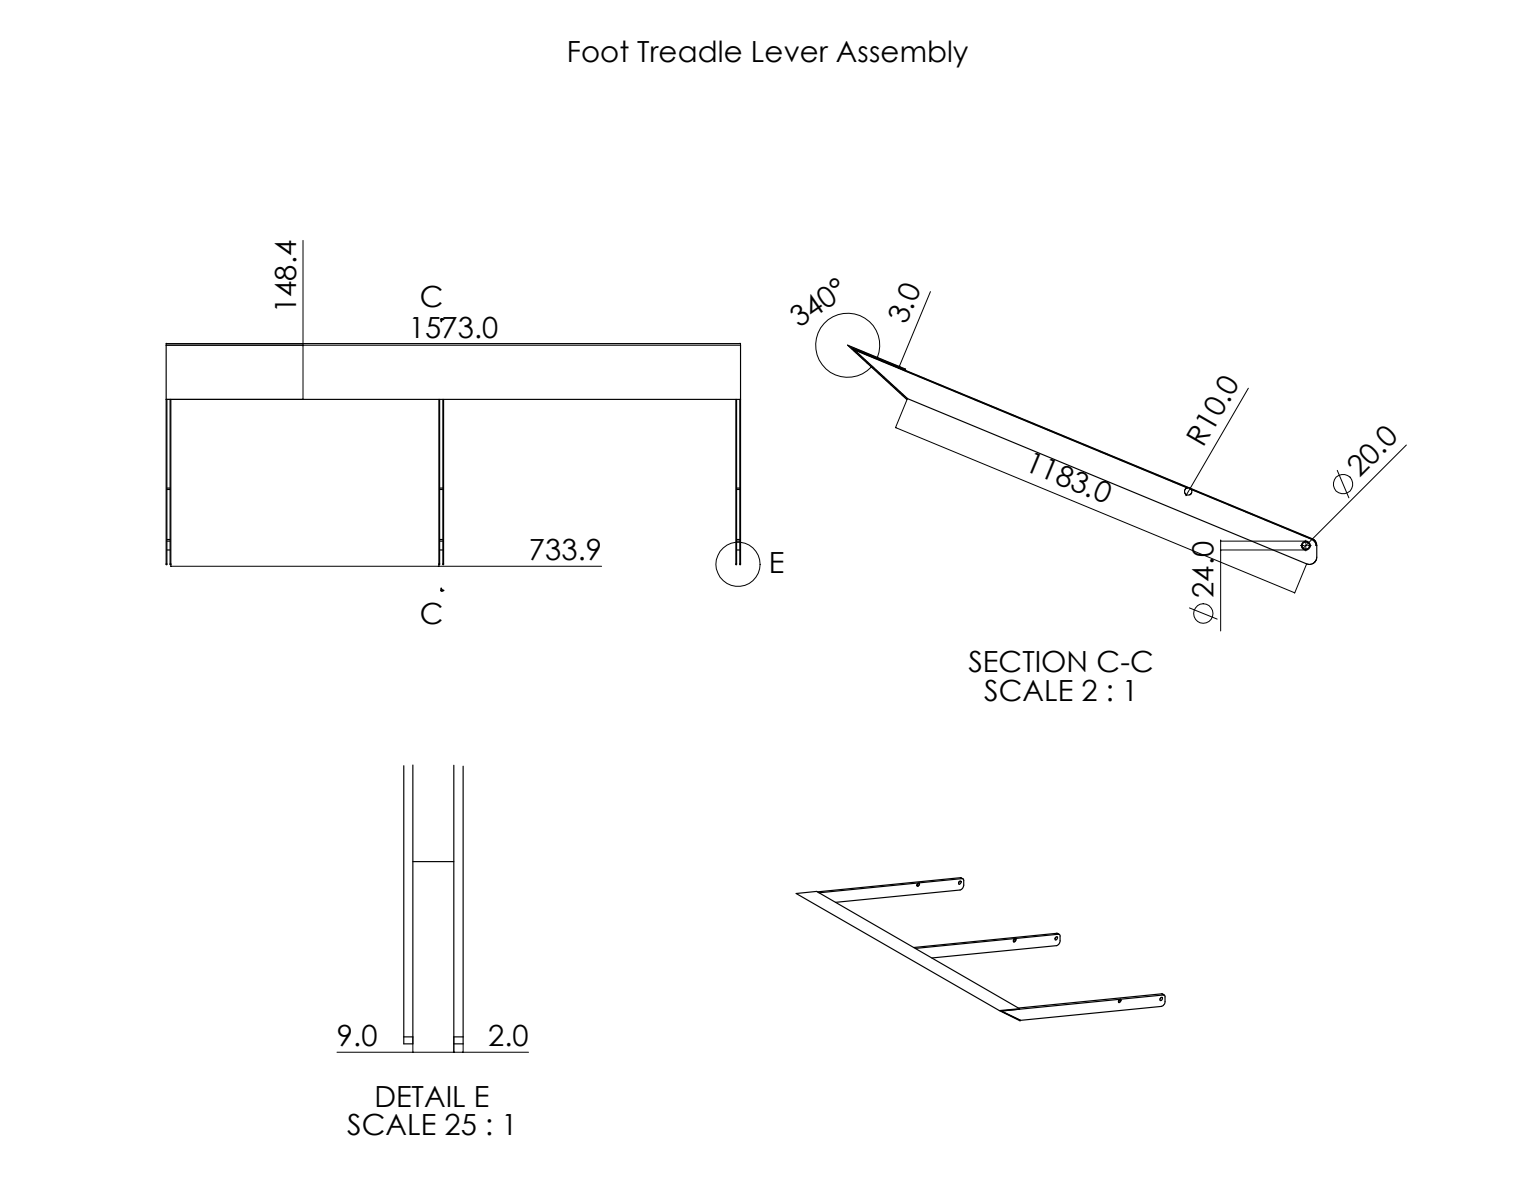
ISO-10303-21;
HEADER;
FILE_DESCRIPTION (('STEP AP214'),
    '1' );
FILE_NAME ('Foot Treadle Lever Assembly.step',
    '2026-10-21T17:07:05',
    ( '' ),
    ( '' ),
    'SwSTEP 2.0',
    'SolidWorks 2025',
    '' );
FILE_SCHEMA (( 'AUTOMOTIVE_DESIGN' ));
ENDSEC;

DATA;
#11=LINE ( 'NONE', #39516, #42666 ) ;
#12=ORIENTED_EDGE ( 'NONE', *, *, #22946, .T. ) ;
#20=ORIENTED_EDGE ( 'NONE', *, *, #3532, .T. ) ;
#69=VERTEX_POINT ( 'NONE', #2595 ) ;
#77=CARTESIAN_POINT ( 'NONE',  ( -39.63011601220123481, -365.3551492539851893, -28.13243251470704109 ) ) ;
#132=EDGE_CURVE ( 'NONE', #43251, #1390, #14358, .T. ) ;
#144=CARTESIAN_POINT ( 'NONE',  ( -786.4999999999993179, -512.9681489794448908, -339.9999999999999432 ) ) ;
#161=LINE ( 'NONE', #18412, #9196 ) ;
#169=EDGE_CURVE ( 'NONE', #1813, #29494, #23376, .T. ) ;
#171=ORIENTED_EDGE ( 'NONE', *, *, #19921, .T. ) ;
#197=CARTESIAN_POINT ( 'NONE',  ( 784.4999999999993179, -513.1383975375929367, -369.9999999999999432 ) ) ;
#209=PLANE ( 'NONE',  #44022 ) ;
#214=AXIS2_PLACEMENT_3D ( 'NONE', #42407, #11013, #31569 ) ;
#235=ORIENTED_EDGE ( 'NONE', *, *, #15168, .F. ) ;
#247=CARTESIAN_POINT ( 'NONE',  ( 775.4999999999993179, -544.8427095258973623, -350.0000000000000000 ) ) ;
#258=VECTOR ( 'NONE', #1525, 1000.000000000000000 ) ;
#260=LINE ( 'NONE', #35579, #37744 ) ;
#292=ORIENTED_EDGE ( 'NONE', *, *, #37389, .F. ) ;
#309=ORIENTED_EDGE ( 'NONE', *, *, #5989, .F. ) ;
#312=FACE_OUTER_BOUND ( 'NONE', #6954, .T. ) ;
#315=DIRECTION ( 'NONE',  ( 0.000000000000000000, 1.000000000000000000, -0.000000000000000000 ) ) ;
#317=EDGE_CURVE ( 'NONE', #3483, #7856, #33327, .T. ) ;
#318=DIRECTION ( 'NONE',  ( 0.000000000000000000, 0.000000000000000000, 1.000000000000000000 ) ) ;
#348=AXIS2_PLACEMENT_3D ( 'NONE', #27817, #38919, #20427 ) ;
#357=ORIENTED_EDGE ( 'NONE', *, *, #4281, .F. ) ;
#384=FACE_OUTER_BOUND ( 'NONE', #6648, .T. ) ;
#385=DIRECTION ( 'NONE',  ( -0.000000000000000000, -0.3826834323650838976, -0.9238795325112892920 ) ) ;
#415=EDGE_LOOP ( 'NONE', ( #32873, #15091, #12065, #25455 ) ) ;
#427=DIRECTION ( 'NONE',  ( 0.000000000000000000, 0.000000000000000000, 1.000000000000000000 ) ) ;
#463=VERTEX_POINT ( 'NONE', #38172 ) ;
#480=EDGE_LOOP ( 'NONE', ( #309, #39907, #31918, #2309 ) ) ;
#501=CARTESIAN_POINT ( 'NONE',  ( -39.63011601220123481, -563.3203001761230553, -342.3463313526983143 ) ) ;
#503=CARTESIAN_POINT ( 'NONE',  ( -773.4999999999993179, -512.9681489794448908, -339.9999999999999432 ) ) ;
#518=VERTEX_POINT ( 'NONE', #16922 ) ;
#526=CARTESIAN_POINT ( 'NONE',  ( 786.4999999999993179, -494.6608068873671300, -357.6536686473015720 ) ) ;
#552=VECTOR ( 'NONE', #9585, 1000.000000000000000 ) ;
#573=CARTESIAN_POINT ( 'NONE',  ( -773.4999999999993179, -365.3551492539851893, -28.13243251470704109 ) ) ;
#598=CARTESIAN_POINT ( 'NONE',  ( -786.4999999999993179, -544.8427095258973623, -350.0000000000000000 ) ) ;
#601=VERTEX_POINT ( 'NONE', #17377 ) ;
#603=CARTESIAN_POINT ( 'NONE',  ( 775.4999999999993179, 22.32581219114657856, 895.6886905569881492 ) ) ;
#611=CARTESIAN_POINT ( 'NONE',  ( 775.4999999999993179, -365.3551492539851893, -18.13243251470705886 ) ) ;
#612=FACE_OUTER_BOUND ( 'NONE', #6643, .T. ) ;
#628=AXIS2_PLACEMENT_3D ( 'NONE', #31793, #14497, #10794 ) ;
#630=PLANE ( 'NONE',  #9977 ) ;
#645=SHAPE_DEFINITION_REPRESENTATION ( #14496, #4721 ) ;
#656=FACE_OUTER_BOUND ( 'NONE', #25655, .T. ) ;
#661=DIRECTION ( 'NONE',  ( -1.000000000000000000, -0.000000000000000000, -0.000000000000000000 ) ) ;
#694=ORIENTED_EDGE ( 'NONE', *, *, #17918, .T. ) ;
#749=ORIENTED_EDGE ( 'NONE', *, *, #32375, .T. ) ;
#757=VERTEX_POINT ( 'NONE', #11595 ) ;
#764=ORIENTED_EDGE ( 'NONE', *, *, #41585, .T. ) ;
#790=DIRECTION ( 'NONE',  ( -1.000000000000000000, -0.000000000000000000, -0.000000000000000000 ) ) ;
#835=CARTESIAN_POINT ( 'NONE',  ( -786.4999999999993179, -544.8427095258973623, -350.0000000000000000 ) ) ;
#842=CYLINDRICAL_SURFACE ( 'NONE', #628, 12.00000000000001066 ) ;
#871=DIRECTION ( 'NONE',  ( 1.000000000000000000, -0.000000000000000000, -0.000000000000000000 ) ) ;
#877=CARTESIAN_POINT ( 'NONE',  ( -37.63011601220122770, -365.3551492539851893, -18.13243251470705886 ) ) ;
#909=CIRCLE ( 'NONE', #14943, 12.00000000000001066 ) ;
#964=VECTOR ( 'NONE', #44223, 999.9999999999998863 ) ;
#968=ORIENTED_EDGE ( 'NONE', *, *, #23222, .T. ) ;
#988=EDGE_CURVE ( 'NONE', #30488, #37811, #44694, .T. ) ;
#993=CARTESIAN_POINT ( 'NONE',  ( -39.63011601220123481, 26.27639943461401018, 900.0000000000001137 ) ) ;
#1012=CYLINDRICAL_SURFACE ( 'NONE', #8516, 19.99999999999990763 ) ;
#1029=VERTEX_POINT ( 'NONE', #23428 ) ;
#1033=VECTOR ( 'NONE', #41918, 1000.000000000000000 ) ;
#1058=CARTESIAN_POINT ( 'NONE',  ( -39.63011601220123481, -513.1383975375929367, -369.9999999999999432 ) ) ;
#1064=CARTESIAN_POINT ( 'NONE',  ( 775.4999999999993179, -544.8427095258973623, -369.9999999999999432 ) ) ;
#1101=PLANE ( 'NONE',  #32125 ) ;
#1103=AXIS2_PLACEMENT_3D ( 'NONE', #14608, #33065, #18972 ) ;
#1111=VERTEX_POINT ( 'NONE', #27142 ) ;
#1114=CARTESIAN_POINT ( 'NONE',  ( 746.4999999999993179, -355.4967352946684969, -16.45562775363632113 ) ) ;
#1131=ADVANCED_FACE ( 'NONE', ( #12811 ), #6108, .T. ) ;
#1132=AXIS2_PLACEMENT_3D ( 'NONE', #28850, #42931, #11297 ) ;
#1138=ORIENTED_EDGE ( 'NONE', *, *, #33206, .F. ) ;
#1159=LINE ( 'NONE', #8320, #2670 ) ;
#1203=AXIS2_PLACEMENT_3D ( 'NONE', #24325, #16957, #10469 ) ;
#1206=ORIENTED_EDGE ( 'NONE', *, *, #37580, .T. ) ;
#1219=ORIENTED_EDGE ( 'NONE', *, *, #41907, .T. ) ;
#1238=AXIS2_PLACEMENT_3D ( 'NONE', #7481, #21783, #18105 ) ;
#1240=LINE ( 'NONE', #4488, #19538 ) ;
#1243=AXIS2_PLACEMENT_3D ( 'NONE', #9404, #29728, #29961 ) ;
#1259=ORIENTED_EDGE ( 'NONE', *, *, #45039, .T. ) ;
#1266=EDGE_CURVE ( 'NONE', #33715, #16430, #19508, .T. ) ;
#1289=FACE_OUTER_BOUND ( 'NONE', #14899, .T. ) ;
#1320=ORIENTED_EDGE ( 'NONE', *, *, #28389, .T. ) ;
#1360=ORIENTED_EDGE ( 'NONE', *, *, #33421, .T. ) ;
#1374=VERTEX_POINT ( 'NONE', #10723 ) ;
#1376=VECTOR ( 'NONE', #35836, 999.9999999999998863 ) ;
#1390=VERTEX_POINT ( 'NONE', #6570 ) ;
#1418=MANIFOLD_SOLID_BREP ( 'Mirror5[3]', #38730 ) ;
#1429=VERTEX_POINT ( 'NONE', #2881 ) ;
#1440=DIRECTION ( 'NONE',  ( 0.000000000000000000, 0.000000000000000000, 1.000000000000000000 ) ) ;
#1480=ORIENTED_EDGE ( 'NONE', *, *, #43372, .T. ) ;
#1487=EDGE_CURVE ( 'NONE', #36764, #29494, #41917, .T. ) ;
#1490=DIRECTION ( 'NONE',  ( 0.000000000000000000, 0.000000000000000000, -1.000000000000000000 ) ) ;
#1499=PLANE ( 'NONE',  #38589 ) ;
#1517=FACE_BOUND ( 'NONE', #4195, .T. ) ;
#1525=DIRECTION ( 'NONE',  ( 1.000000000000000000, -0.000000000000000000, -0.000000000000000000 ) ) ;
#1530=ADVANCED_FACE ( 'NONE', ( #14425 ), #42133, .F. ) ;
#1535=ORIENTED_EDGE ( 'NONE', *, *, #32375, .F. ) ;
#1556=ORIENTED_EDGE ( 'NONE', *, *, #21278, .F. ) ;
#1559=DIRECTION ( 'NONE',  ( 1.000000000000000000, 0.000000000000000000, -0.000000000000000000 ) ) ;
#1640=ORIENTED_EDGE ( 'NONE', *, *, #30606, .T. ) ;
#1655=LINE ( 'NONE', #33102, #38693 ) ;
#1705=CIRCLE ( 'NONE', #44413, 12.00000000000001066 ) ;
#1718=CARTESIAN_POINT ( 'NONE',  ( 773.4999999999993179, -110.5936016518799221, 750.6326042729449455 ) ) ;
#1734=ORIENTED_EDGE ( 'NONE', *, *, #8319, .T. ) ;
#1743=ORIENTED_EDGE ( 'NONE', *, *, #15407, .F. ) ;
#1755=DIRECTION ( 'NONE',  ( 0.000000000000000000, 0.7372773368101328550, -0.6755902076156506952 ) ) ;
#1763=DIRECTION ( 'NONE',  ( -1.000000000000000000, -0.000000000000000000, -0.000000000000000000 ) ) ;
#1776=EDGE_CURVE ( 'NONE', #14297, #8747, #14884, .T. ) ;
#1795=ORIENTED_EDGE ( 'NONE', *, *, #40528, .F. ) ;
#1800=DIRECTION ( 'NONE',  ( 0.000000000000000000, 0.3826834323650836756, 0.9238795325112892920 ) ) ;
#1813=VERTEX_POINT ( 'NONE', #33115 ) ;
#1816=ORIENTED_EDGE ( 'NONE', *, *, #41907, .F. ) ;
#1833=CARTESIAN_POINT ( 'NONE',  ( -786.4999999999993179, -365.3551492539851893, -8.132432514707076621 ) ) ;
#1867=ORIENTED_EDGE ( 'NONE', *, *, #39030, .T. ) ;
#1888=DIRECTION ( 'NONE',  ( 0.000000000000000000, 0.3826834323650836756, 0.9238795325112892920 ) ) ;
#1893=VECTOR ( 'NONE', #35927, 1000.000000000000114 ) ;
#1895=DIRECTION ( 'NONE',  ( 0.000000000000000000, 0.000000000000000000, 1.000000000000000000 ) ) ;
#1921=ORIENTED_EDGE ( 'NONE', *, *, #37141, .F. ) ;
#1923=VECTOR ( 'NONE', #5270, 1000.000000000000114 ) ;
#1925=( NAMED_UNIT ( * ) SI_UNIT ( $, .STERADIAN. ) SOLID_ANGLE_UNIT ( ) );
#1926=AXIS2_PLACEMENT_3D ( 'NONE', #2058, #12918, #37160 ) ;
#1959=DIRECTION ( 'NONE',  ( 0.000000000000000000, -0.3826834323650836756, -0.9238795325112892920 ) ) ;
#1991=AXIS2_PLACEMENT_3D ( 'NONE', #31297, #3813, #21817 ) ;
#1996=CIRCLE ( 'NONE', #10121, 9.999999999999982236 ) ;
#1998=DIRECTION ( 'NONE',  ( 1.000000000000000000, 0.000000000000000000, -0.000000000000000000 ) ) ;
#2008=CARTESIAN_POINT ( 'NONE',  ( -28.63011601220122415, -501.1515549466498669, -368.0974687824633520 ) ) ;
#2030=ADVANCED_FACE ( 'NONE', ( #37471 ), #16221, .F. ) ;
#2041=ORIENTED_EDGE ( 'NONE', *, *, #11895, .F. ) ;
#2056=AXIS2_PLACEMENT_3D ( 'NONE', #19204, #36975, #15306 ) ;
#2058=CARTESIAN_POINT ( 'NONE',  ( -786.4999999999993179, -512.9681489794448908, -339.9999999999999432 ) ) ;
#2064=VERTEX_POINT ( 'NONE', #22914 ) ;
#2085=ADVANCED_FACE ( 'NONE', ( #40494 ), #20136, .T. ) ;
#2103=VERTEX_POINT ( 'NONE', #5150 ) ;
#2118=DIRECTION ( 'NONE',  ( 0.000000000000000000, 0.000000000000000000, -1.000000000000000000 ) ) ;
#2163=EDGE_LOOP ( 'NONE', ( #2260, #40842 ) ) ;
#2171=VERTEX_POINT ( 'NONE', #27982 ) ;
#2173=FACE_OUTER_BOUND ( 'NONE', #43522, .T. ) ;
#2175=EDGE_LOOP ( 'NONE', ( #2685, #9652 ) ) ;
#2190=DIRECTION ( 'NONE',  ( -1.000000000000000000, -0.000000000000000000, -0.000000000000000000 ) ) ;
#2212=ORIENTED_EDGE ( 'NONE', *, *, #10099, .F. ) ;
#2217=ORIENTED_EDGE ( 'NONE', *, *, #15681, .F. ) ;
#2219=ORIENTED_EDGE ( 'NONE', *, *, #36874, .F. ) ;
#2247=ORIENTED_EDGE ( 'NONE', *, *, #26936, .F. ) ;
#2257=CARTESIAN_POINT ( 'NONE',  ( -28.63011601220122415, -857.0166862835568509, -63.94525337997358605 ) ) ;
#2260=ORIENTED_EDGE ( 'NONE', *, *, #28130, .F. ) ;
#2273=VERTEX_POINT ( 'NONE', #44865 ) ;
#2291=LINE ( 'NONE', #22859, #8243 ) ;
#2309=ORIENTED_EDGE ( 'NONE', *, *, #15175, .T. ) ;
#2313=EDGE_CURVE ( 'NONE', #30501, #26595, #11394, .T. ) ;
#2326=ORIENTED_EDGE ( 'NONE', *, *, #36268, .T. ) ;
#2367=EDGE_CURVE ( 'NONE', #2677, #39212, #37185, .T. ) ;
#2381=EDGE_LOOP ( 'NONE', ( #23102, #23854, #14000, #2217, #1867, #3901, #27773, #25609, #12738, #13022, #39635, #33451 ) ) ;
#2388=CARTESIAN_POINT ( 'NONE',  ( 786.4999999999993179, -512.9681489794448908, -339.9999999999999432 ) ) ;
#2391=EDGE_LOOP ( 'NONE', ( #6090, #18144, #8044, #23562 ) ) ;
#2408=CARTESIAN_POINT ( 'NONE',  ( -66.63011601220125613, -359.5698779088871788, -26.28906389436294688 ) ) ;
#2413=DIRECTION ( 'NONE',  ( 1.000000000000000000, -0.000000000000000000, -0.000000000000000000 ) ) ;
#2426=CARTESIAN_POINT ( 'NONE',  ( -26.63011601220122060, -544.8427095258973623, -369.9999999999999432 ) ) ;
#2442=CIRCLE ( 'NONE', #9836, 9.999999999999980460 ) ;
#2451=CARTESIAN_POINT ( 'NONE',  ( 784.4999999999993179, -544.8427095258973623, -369.9999999999999432 ) ) ;
#2460=CARTESIAN_POINT ( 'NONE',  ( 773.4999999999993179, -513.1383975375929367, -369.9999999999999432 ) ) ;
#2463=LINE ( 'NONE', #29964, #24876 ) ;
#2472=DIRECTION ( 'NONE',  ( -1.000000000000000000, -0.000000000000000000, -0.000000000000000000 ) ) ;
#2475=AXIS2_PLACEMENT_3D ( 'NONE', #835, #35477, #7779 ) ;
#2495=VERTEX_POINT ( 'NONE', #18057 ) ;
#2505=AXIS2_PLACEMENT_3D ( 'NONE', #7274, #13509, #10484 ) ;
#2507=ORIENTED_EDGE ( 'NONE', *, *, #20142, .T. ) ;
#2526=AXIS2_PLACEMENT_3D ( 'NONE', #30837, #37766, #6115 ) ;
#2529=FACE_OUTER_BOUND ( 'NONE', #15063, .T. ) ;
#2561=ORIENTED_EDGE ( 'NONE', *, *, #11429, .F. ) ;
#2587=CARTESIAN_POINT ( 'NONE',  ( 1007.605605532488426, -295.7697417039441916, 122.5118383533586837 ) ) ;
#2590=DIRECTION ( 'NONE',  ( 0.000000000000000000, 0.000000000000000000, -1.000000000000000000 ) ) ;
#2595=CARTESIAN_POINT ( 'NONE',  ( -773.4999999999993179, -563.3203001761230553, -342.3463313526983143 ) ) ;
#2609=CIRCLE ( 'NONE', #10002, 9.999999999999982236 ) ;
#2614=VECTOR ( 'NONE', #34560, 1000.000000000000000 ) ;
#2615=ORIENTED_EDGE ( 'NONE', *, *, #30089, .T. ) ;
#2634=LINE ( 'NONE', #19962, #23991 ) ;
#2635=DIRECTION ( 'NONE',  ( -1.000000000000000000, -0.000000000000000000, 0.000000000000000000 ) ) ;
#2651=CARTESIAN_POINT ( 'NONE',  ( -773.4999999999993179, -513.1383975375929367, -349.9999999999999432 ) ) ;
#2670=VECTOR ( 'NONE', #22384, 1000.000000000000114 ) ;
#2677=VERTEX_POINT ( 'NONE', #21737 ) ;
#2685=ORIENTED_EDGE ( 'NONE', *, *, #32862, .T. ) ;
#2700=FACE_OUTER_BOUND ( 'NONE', #35564, .T. ) ;
#2708=EDGE_CURVE ( 'NONE', #5066, #9279, #9897, .T. ) ;
#2716=CARTESIAN_POINT ( 'NONE',  ( -37.63011601220122770, -544.8427095258973623, -350.0000000000000000 ) ) ;
#2731=CIRCLE ( 'NONE', #18210, 10.00000000000000888 ) ;
#2753=CIRCLE ( 'NONE', #18985, 10.00000000000000888 ) ;
#2796=CARTESIAN_POINT ( 'NONE',  ( -26.63011601220122060, -110.5936016518799221, 750.6326042729449455 ) ) ;
#2824=DIRECTION ( 'NONE',  ( -1.000000000000000000, -0.000000000000000000, 0.000000000000000000 ) ) ;
#2847=ORIENTED_EDGE ( 'NONE', *, *, #24646, .T. ) ;
#2856=CIRCLE ( 'NONE', #24244, 9.999999999999980460 ) ;
#2863=ORIENTED_EDGE ( 'NONE', *, *, #5989, .T. ) ;
#2866=CARTESIAN_POINT ( 'NONE',  ( 746.4999999999993179, -365.3551492539851893, -8.132432514707076621 ) ) ;
#2875=CARTESIAN_POINT ( 'NONE',  ( -775.4999999999993179, -365.3551492539851893, -18.13243251470705886 ) ) ;
#2881=CARTESIAN_POINT ( 'NONE',  ( 775.4999999999993179, -563.3203001761230553, -342.3463313526983143 ) ) ;
#2892=CIRCLE ( 'NONE', #14720, 12.00000000000001066 ) ;
#2897=ORIENTED_EDGE ( 'NONE', *, *, #38295, .F. ) ;
#2902=CARTESIAN_POINT ( 'NONE',  ( 786.4999999999993179, -496.5085659523897448, -356.8883017825714319 ) ) ;
#2912=ORIENTED_EDGE ( 'NONE', *, *, #37065, .T. ) ;
#2918=CARTESIAN_POINT ( 'NONE',  ( -26.63011601220122060, -512.9681489794448908, -352.0000000000000000 ) ) ;
#2932=DIRECTION ( 'NONE',  ( -0.000000000000000000, 1.000000000000000000, -0.000000000000000000 ) ) ;
#2937=CARTESIAN_POINT ( 'NONE',  ( 786.4999999999993179, -365.3551492539851893, -8.132432514707076621 ) ) ;
#2943=ORIENTED_EDGE ( 'NONE', *, *, #32872, .T. ) ;
#2947=EDGE_CURVE ( 'NONE', #11840, #5018, #12035, .T. ) ;
#2950=CARTESIAN_POINT ( 'NONE',  ( -786.4999999999993179, -494.6608068873671300, -357.6536686473015720 ) ) ;
#2955=CARTESIAN_POINT ( 'NONE',  ( -39.63011601220123481, -512.9681489794448908, -339.9999999999999432 ) ) ;
#2958=VERTEX_POINT ( 'NONE', #33493 ) ;
#3021=LINE ( 'NONE', #2796, #39689 ) ;
#3085=DIRECTION ( 'NONE',  ( 1.000000000000000000, 0.000000000000000000, -0.000000000000000000 ) ) ;
#3086=LINE ( 'NONE', #2866, #40334 ) ;
#3089=VECTOR ( 'NONE', #24966, 1000.000000000000000 ) ;
#3121=FACE_OUTER_BOUND ( 'NONE', #37828, .T. ) ;
#3143=AXIS2_PLACEMENT_3D ( 'NONE', #45436, #38276, #45669 ) ;
#3146=CYLINDRICAL_SURFACE ( 'NONE', #3469, 10.00000000000000888 ) ;
#3152=DIRECTION ( 'NONE',  ( -1.000000000000000000, -0.000000000000000000, -0.000000000000000000 ) ) ;
#3157=DIRECTION ( 'NONE',  ( -1.000000000000000000, -0.000000000000000000, -0.000000000000000000 ) ) ;
#3169=DIRECTION ( 'NONE',  ( -1.000000000000000000, 0.000000000000000000, 0.000000000000000000 ) ) ;
#3174=DIRECTION ( 'NONE',  ( 0.000000000000000000, 0.000000000000000000, -1.000000000000000000 ) ) ;
#3186=ORIENTED_EDGE ( 'NONE', *, *, #45316, .T. ) ;
#3187=AXIS2_PLACEMENT_3D ( 'NONE', #13354, #45692, #3174 ) ;
#3201=CARTESIAN_POINT ( 'NONE',  ( 786.4999999999993179, -544.8427095258973623, -369.9999999999999432 ) ) ;
#3219=CIRCLE ( 'NONE', #24604, 18.00000000000001421 ) ;
#3263=DIRECTION ( 'NONE',  ( -1.000000000000000000, -0.000000000000000000, 0.000000000000000000 ) ) ;
#3293=ORIENTED_EDGE ( 'NONE', *, *, #27744, .F. ) ;
#3312=ORIENTED_EDGE ( 'NONE', *, *, #8604, .F. ) ;
#3315=AXIS2_PLACEMENT_3D ( 'NONE', #45042, #34639, #16633 ) ;
#3320=MANIFOLD_SOLID_BREP ( 'Cut-Extrude8', #6229 ) ;
#3337=AXIS2_PLACEMENT_3D ( 'NONE', #41849, #38377, #14122 ) ;
#3342=( NAMED_UNIT ( * ) PLANE_ANGLE_UNIT ( ) SI_UNIT ( $, .RADIAN. ) );
#3376=ORIENTED_EDGE ( 'NONE', *, *, #23841, .T. ) ;
#3451=AXIS2_PLACEMENT_3D ( 'NONE', #42334, #21326, #31709 ) ;
#3469=AXIS2_PLACEMENT_3D ( 'NONE', #144, #6618, #38485 ) ;
#3483=VERTEX_POINT ( 'NONE', #18684 ) ;
#3497=CARTESIAN_POINT ( 'NONE',  ( -786.4999999999993179, -110.5936016518799221, 750.6326042729449455 ) ) ;
#3499=DIRECTION ( 'NONE',  ( 1.000000000000000000, 0.000000000000000000, -0.000000000000000000 ) ) ;
#3511=DIRECTION ( 'NONE',  ( 0.000000000000000000, 0.000000000000000000, -1.000000000000000000 ) ) ;
#3517=DIRECTION ( 'NONE',  ( 0.000000000000000000, 0.000000000000000000, 1.000000000000000000 ) ) ;
#3532=EDGE_CURVE ( 'NONE', #35031, #33715, #11535, .T. ) ;
#3533=CARTESIAN_POINT ( 'NONE',  ( -786.4999999999993179, -513.1383975375929367, -369.9999999999999432 ) ) ;
#3542=VERTEX_POINT ( 'NONE', #21927 ) ;
#3545=PLANE ( 'NONE',  #24184 ) ;
#3550=ADVANCED_FACE ( 'NONE', ( #25617 ), #32324, .T. ) ;
#3561=DIRECTION ( 'NONE',  ( 1.000000000000000000, -0.000000000000000000, -0.000000000000000000 ) ) ;
#3601=CARTESIAN_POINT ( 'NONE',  ( -28.63011601220122415, -563.3203001761231690, -342.3463313526983143 ) ) ;
#3612=VERTEX_POINT ( 'NONE', #23552 ) ;
#3616=DIRECTION ( 'NONE',  ( 0.000000000000000000, 0.000000000000000000, 1.000000000000000000 ) ) ;
#3642=CARTESIAN_POINT ( 'NONE',  ( -26.63011601220122060, -365.3551492539851893, -8.132432514707076621 ) ) ;
#3648=LINE ( 'NONE', #7110, #17334 ) ;
#3705=ORIENTED_EDGE ( 'NONE', *, *, #17646, .F. ) ;
#3726=ORIENTED_EDGE ( 'NONE', *, *, #27806, .F. ) ;
#3741=CARTESIAN_POINT ( 'NONE',  ( -37.63011601220122770, -512.9681489794448908, -352.0000000000000000 ) ) ;
#3768=ORIENTED_EDGE ( 'NONE', *, *, #28665, .F. ) ;
#3776=ORIENTED_EDGE ( 'NONE', *, *, #45342, .T. ) ;
#3799=EDGE_CURVE ( 'NONE', #36535, #14349, #2609, .T. ) ;
#3800=LINE ( 'NONE', #28968, #14383 ) ;
#3809=ORIENTED_EDGE ( 'NONE', *, *, #12744, .F. ) ;
#3813=DIRECTION ( 'NONE',  ( -1.000000000000000000, 0.000000000000000000, 0.000000000000000000 ) ) ;
#3818=ADVANCED_FACE ( 'NONE', ( #40894 ), #12490, .F. ) ;
#3837=CARTESIAN_POINT ( 'NONE',  ( -784.4999999999993179, -544.8427095258973623, -350.0000000000000000 ) ) ;
#3860=CARTESIAN_POINT ( 'NONE',  ( -784.4999999999993179, -365.3551492539851893, -18.13243251470705886 ) ) ;
#3870=CYLINDRICAL_SURFACE ( 'NONE', #3187, 9.999999999999980460 ) ;
#3876=VECTOR ( 'NONE', #8066, 1000.000000000000000 ) ;
#3891=DIRECTION ( 'NONE',  ( 0.000000000000000000, 0.000000000000000000, 1.000000000000000000 ) ) ;
#3901=ORIENTED_EDGE ( 'NONE', *, *, #6862, .T. ) ;
#3941=VECTOR ( 'NONE', #43200, 1000.000000000000000 ) ;
#3965=CARTESIAN_POINT ( 'NONE',  ( 786.4999999999993179, -544.8427095258973623, -369.9999999999999432 ) ) ;
#4005=FACE_OUTER_BOUND ( 'NONE', #18702, .T. ) ;
#4006=AXIS2_PLACEMENT_3D ( 'NONE', #9807, #34741, #34279 ) ;
#4041=VECTOR ( 'NONE', #22643, 1000.000000000000114 ) ;
#4047=VECTOR ( 'NONE', #8844, 1000.000000000000000 ) ;
#4067=VERTEX_POINT ( 'NONE', #29061 ) ;
#4073=CARTESIAN_POINT ( 'NONE',  ( 746.4999999999993179, -365.3551492539851893, -18.13243251470705886 ) ) ;
#4084=ADVANCED_FACE ( 'NONE', ( #10827, #656, #18227 ), #25354, .F. ) ;
#4119=VECTOR ( 'NONE', #8933, 1000.000000000000000 ) ;
#4136=CIRCLE ( 'NONE', #36560, 12.00000000000001066 ) ;
#4161=VECTOR ( 'NONE', #30084, 1000.000000000000114 ) ;
#4169=ADVANCED_FACE ( 'NONE', ( #32754 ), #1101, .T. ) ;
#4186=ORIENTED_EDGE ( 'NONE', *, *, #41613, .F. ) ;
#4195=EDGE_LOOP ( 'NONE', ( #34713, #2219 ) ) ;
#4226=ORIENTED_EDGE ( 'NONE', *, *, #132, .T. ) ;
#4245=ORIENTED_EDGE ( 'NONE', *, *, #4281, .T. ) ;
#4270=DIRECTION ( 'NONE',  ( -1.000000000000000000, -0.000000000000000000, -0.000000000000000000 ) ) ;
#4271=ORIENTED_EDGE ( 'NONE', *, *, #20771, .T. ) ;
#4275=DIRECTION ( 'NONE',  ( 1.000000000000000000, -0.000000000000000000, -0.000000000000000000 ) ) ;
#4281=EDGE_CURVE ( 'NONE', #33261, #44892, #11744, .T. ) ;
#4297=CARTESIAN_POINT ( 'NONE',  ( 773.4999999999993179, -544.8427095258973623, -369.9999999999999432 ) ) ;
#4300=ORIENTED_EDGE ( 'NONE', *, *, #37389, .T. ) ;
#4309=LINE ( 'NONE', #11695, #44390 ) ;
#4320=EDGE_CURVE ( 'NONE', #14349, #36535, #20311, .T. ) ;
#4326=AXIS2_PLACEMENT_3D ( 'NONE', #28800, #38984, #43109 ) ;
#4358=VERTEX_POINT ( 'NONE', #23170 ) ;
#4382=ORIENTED_EDGE ( 'NONE', *, *, #14505, .T. ) ;
#4397=CARTESIAN_POINT ( 'NONE',  ( -786.4999999999993179, -496.5085659523897448, -356.8883017825714319 ) ) ;
#4398=ADVANCED_FACE ( 'NONE', ( #2173 ), #18900, .F. ) ;
#4401=EDGE_CURVE ( 'NONE', #13363, #45720, #2634, .T. ) ;
#4428=EDGE_CURVE ( 'NONE', #44892, #44015, #21080, .T. ) ;
#4454=VERTEX_POINT ( 'NONE', #37972 ) ;
#4467=CARTESIAN_POINT ( 'NONE',  ( 786.4999999999993179, 262.9227088301245203, 634.7515695135432452 ) ) ;
#4488=CARTESIAN_POINT ( 'NONE',  ( 786.4999999999993179, -110.5936016518799221, 750.6326042729449455 ) ) ;
#4529=FACE_OUTER_BOUND ( 'NONE', #29351, .T. ) ;
#4544=DIRECTION ( 'NONE',  ( -1.000000000000000000, -0.000000000000000000, -0.000000000000000000 ) ) ;
#4571=CARTESIAN_POINT ( 'NONE',  ( 775.4999999999993179, -365.3551492539851893, -28.13243251470704109 ) ) ;
#4577=DIRECTION ( 'NONE',  ( 1.000000000000000000, -0.000000000000000000, -0.000000000000000000 ) ) ;
#4580=LINE ( 'NONE', #26498, #3876 ) ;
#4607=ORIENTED_EDGE ( 'NONE', *, *, #43372, .F. ) ;
#4634=CARTESIAN_POINT ( 'NONE',  ( -26.63011601220122060, -513.1383975375929367, -349.9999999999999432 ) ) ;
#4642=EDGE_CURVE ( 'NONE', #6318, #39517, #7809, .T. ) ;
#4667=ORIENTED_EDGE ( 'NONE', *, *, #6862, .F. ) ;
#4703=VERTEX_POINT ( 'NONE', #24544 ) ;
#4721=SHAPE_REPRESENTATION ( 'Foot Treadle Lever Assembly', ( #26858 ), #34210 ) ;
#4722=EDGE_CURVE ( 'NONE', #42387, #22673, #38657, .T. ) ;
#4751=VECTOR ( 'NONE', #28100, 1000.000000000000000 ) ;
#4811=DIRECTION ( 'NONE',  ( 1.000000000000000000, -0.000000000000000000, -0.000000000000000000 ) ) ;
#4851=EDGE_LOOP ( 'NONE', ( #36463, #27555, #7077, #13940, #1219, #41795, #40284, #31017, #25069, #41649, #42787 ) ) ;
#4854=CARTESIAN_POINT ( 'NONE',  ( -66.63011601220125613, -365.3551492539851893, -18.13243251470705886 ) ) ;
#4891=EDGE_CURVE ( 'NONE', #1429, #37268, #16571, .T. ) ;
#4897=CIRCLE ( 'NONE', #14513, 9.999999999999982236 ) ;
#4914=ORIENTED_EDGE ( 'NONE', *, *, #13446, .T. ) ;
#4922=DIRECTION ( 'NONE',  ( 1.000000000000000000, 0.000000000000000000, -0.000000000000000000 ) ) ;
#4943=ORIENTED_EDGE ( 'NONE', *, *, #11926, .F. ) ;
#4962=VECTOR ( 'NONE', #41227, 1000.000000000000000 ) ;
#4980=DIRECTION ( 'NONE',  ( -1.000000000000000000, 0.000000000000000000, 0.000000000000000000 ) ) ;
#4988=ADVANCED_FACE ( 'NONE', ( #39819 ), #29407, .T. ) ;
#5012=AXIS2_PLACEMENT_3D ( 'NONE', #28929, #32405, #10686 ) ;
#5018=VERTEX_POINT ( 'NONE', #43479 ) ;
#5026=CARTESIAN_POINT ( 'NONE',  ( -786.4999999999993179, -512.9681489794448908, -329.9999999999999432 ) ) ;
#5056=CARTESIAN_POINT ( 'NONE',  ( 784.4999999999993179, -513.1383975375929367, -369.9999999999999432 ) ) ;
#5066=VERTEX_POINT ( 'NONE', #11847 ) ;
#5075=EDGE_LOOP ( 'NONE', ( #31549, #6184 ) ) ;
#5117=VERTEX_POINT ( 'NONE', #43700 ) ;
#5134=FACE_OUTER_BOUND ( 'NONE', #13937, .T. ) ;
#5150=CARTESIAN_POINT ( 'NONE',  ( -784.4999999999993179, -110.5936016518799221, 750.6326042729449455 ) ) ;
#5168=CARTESIAN_POINT ( 'NONE',  ( -37.63011601220122770, -496.5085659523897448, -356.8883017825714319 ) ) ;
#5182=EDGE_CURVE ( 'NONE', #36107, #601, #1655, .T. ) ;
#5248=LINE ( 'NONE', #40597, #11606 ) ;
#5270=DIRECTION ( 'NONE',  ( 0.000000000000000000, -0.6755902076156505842, -0.7372773368101327440 ) ) ;
#5337=EDGE_LOOP ( 'NONE', ( #40422, #292, #10993, #45248 ) ) ;
#5372=DIRECTION ( 'NONE',  ( -1.000000000000000000, -0.000000000000000000, -0.000000000000000000 ) ) ;
#5398=AXIS2_PLACEMENT_3D ( 'NONE', #4634, #6787, #18294 ) ;
#5426=CARTESIAN_POINT ( 'NONE',  ( -773.4999999999993179, -544.8427095258973623, -350.0000000000000000 ) ) ;
#5437=( NAMED_UNIT ( * ) PLANE_ANGLE_UNIT ( ) SI_UNIT ( $, .RADIAN. ) );
#5450=AXIS2_PLACEMENT_3D ( 'NONE', #19014, #12077, #36561 ) ;
#5518=ADVANCED_FACE ( 'NONE', ( #24914, #42024 ), #209, .T. ) ;
#5538=AXIS2_PLACEMENT_3D ( 'NONE', #14758, #21906, #427 ) ;
#5564=ORIENTED_EDGE ( 'NONE', *, *, #13446, .F. ) ;
#5577=ORIENTED_EDGE ( 'NONE', *, *, #10584, .T. ) ;
#5622=ORIENTED_EDGE ( 'NONE', *, *, #37385, .F. ) ;
#5655=LINE ( 'NONE', #2408, #22653 ) ;
#5658=CARTESIAN_POINT ( 'NONE',  ( -26.63011601220122060, -494.6608068873671300, -357.6536686473015720 ) ) ;
#5670=LINE ( 'NONE', #22978, #25449 ) ;
#5674=ORIENTED_EDGE ( 'NONE', *, *, #11458, .T. ) ;
#5708=FACE_OUTER_BOUND ( 'NONE', #31644, .T. ) ;
#5751=ORIENTED_EDGE ( 'NONE', *, *, #32627, .T. ) ;
#5782=LINE ( 'NONE', #16639, #13979 ) ;
#5817=EDGE_CURVE ( 'NONE', #4454, #22673, #29528, .T. ) ;
#5821=EDGE_CURVE ( 'NONE', #24190, #26595, #11969, .T. ) ;
#5831=CARTESIAN_POINT ( 'NONE',  ( -773.4999999999993179, -110.5936016518799221, 750.6326042729449455 ) ) ;
#5833=CARTESIAN_POINT ( 'NONE',  ( -26.63011601220122060, -494.6608068873671300, -357.6536686473015720 ) ) ;
#5836=CARTESIAN_POINT ( 'NONE',  ( 784.4999999999993179, 22.32581219114657856, 895.6886905569881492 ) ) ;
#5862=ORIENTED_EDGE ( 'NONE', *, *, #317, .T. ) ;
#5867=LINE ( 'NONE', #18037, #45475 ) ;
#5868=CARTESIAN_POINT ( 'NONE',  ( 773.4999999999993179, -513.1383975375929367, -349.9999999999999432 ) ) ;
#5872=CARTESIAN_POINT ( 'NONE',  ( -786.4999999999993179, -513.1383975375929367, -349.9999999999999432 ) ) ;
#5874=ORIENTED_EDGE ( 'NONE', *, *, #28330, .T. ) ;
#5877=DIRECTION ( 'NONE',  ( 0.000000000000000000, 0.3826834323650836756, 0.9238795325112892920 ) ) ;
#5915=EDGE_LOOP ( 'NONE', ( #33444, #35634, #11438, #18589 ) ) ;
#5927=DIRECTION ( 'NONE',  ( 0.000000000000000000, 1.000000000000000000, -0.000000000000000000 ) ) ;
#5936=CARTESIAN_POINT ( 'NONE',  ( 786.4999999999993179, -512.9681489794448908, -339.9999999999999432 ) ) ;
#5989=EDGE_CURVE ( 'NONE', #30700, #15113, #5655, .T. ) ;
#6009=EDGE_CURVE ( 'NONE', #17287, #23251, #2753, .T. ) ;
#6032=CARTESIAN_POINT ( 'NONE',  ( 784.4999999999993179, -365.3551492539851893, -28.13243251470704109 ) ) ;
#6053=DIRECTION ( 'NONE',  ( 0.000000000000000000, 0.000000000000000000, 1.000000000000000000 ) ) ;
#6060=EDGE_CURVE ( 'NONE', #22319, #19543, #16279, .T. ) ;
#6065=ADVANCED_FACE ( 'NONE', ( #23425 ), #30358, .F. ) ;
#6075=DIRECTION ( 'NONE',  ( 1.000000000000000000, 0.000000000000000000, 0.000000000000000000 ) ) ;
#6090=ORIENTED_EDGE ( 'NONE', *, *, #23320, .F. ) ;
#6101=CARTESIAN_POINT ( 'NONE',  ( -786.4999999999993179, -295.7697417039441916, 122.5118383533586837 ) ) ;
#6108=CYLINDRICAL_SURFACE ( 'NONE', #26110, 12.00000000000001066 ) ;
#6115=DIRECTION ( 'NONE',  ( 0.000000000000000000, 0.000000000000000000, 1.000000000000000000 ) ) ;
#6119=DIRECTION ( 'NONE',  ( -1.000000000000000000, 0.000000000000000000, 0.000000000000000000 ) ) ;
#6130=ORIENTED_EDGE ( 'NONE', *, *, #32264, .F. ) ;
#6138=ORIENTED_EDGE ( 'NONE', *, *, #35330, .F. ) ;
#6184=ORIENTED_EDGE ( 'NONE', *, *, #26462, .T. ) ;
#6229=CLOSED_SHELL ( 'NONE', ( #10346, #12867, #37117, #1530, #18516, #8801, #36126, #7214, #32583, #4084, #43045, #19268, #33761, #23580, #4988, #36322, #44499, #16813, #16830, #24365, #43560, #33510, #24320, #12302 ) ) ;
#6238=ORIENTED_EDGE ( 'NONE', *, *, #27806, .T. ) ;
#6241=UNCERTAINTY_MEASURE_WITH_UNIT (LENGTH_MEASURE( 1.000000000000000082E-05 ), #45148, 'distance_accuracy_value', 'NONE');
#6260=ORIENTED_EDGE ( 'NONE', *, *, #33421, .F. ) ;
#6276=ADVANCED_FACE ( 'NONE', ( #42130 ), #13506, .T. ) ;
#6318=VERTEX_POINT ( 'NONE', #17432 ) ;
#6342=EDGE_CURVE ( 'NONE', #4067, #1813, #42351, .T. ) ;
#6349=VECTOR ( 'NONE', #44431, 1000.000000000000000 ) ;
#6367=VECTOR ( 'NONE', #21963, 1000.000000000000000 ) ;
#6385=CIRCLE ( 'NONE', #3451, 19.99999999999990763 ) ;
#6481=ORIENTED_EDGE ( 'NONE', *, *, #37385, .T. ) ;
#6498=ORIENTED_EDGE ( 'NONE', *, *, #25485, .T. ) ;
#6503=ORIENTED_EDGE ( 'NONE', *, *, #10845, .T. ) ;
#6538=EDGE_LOOP ( 'NONE', ( #4300, #10500 ) ) ;
#6553=ORIENTED_EDGE ( 'NONE', *, *, #11895, .T. ) ;
#6570=CARTESIAN_POINT ( 'NONE',  ( -784.4999999999993179, -512.9681489794448908, -352.0000000000000000 ) ) ;
#6611=EDGE_CURVE ( 'NONE', #14349, #38546, #21561, .T. ) ;
#6618=DIRECTION ( 'NONE',  ( 1.000000000000000000, -0.000000000000000000, -0.000000000000000000 ) ) ;
#6633=DIRECTION ( 'NONE',  ( 0.000000000000000000, 0.3826834323650838421, 0.9238795325112891810 ) ) ;
#6641=DIRECTION ( 'NONE',  ( 0.000000000000000000, 0.000000000000000000, -1.000000000000000000 ) ) ;
#6643=EDGE_LOOP ( 'NONE', ( #35857, #18885, #44425, #10145 ) ) ;
#6648=EDGE_LOOP ( 'NONE', ( #32461, #24761, #13432, #33753 ) ) ;
#6670=CARTESIAN_POINT ( 'NONE',  ( 786.4999999999993179, -563.3203001761230553, -342.3463313526983143 ) ) ;
#6699=EDGE_LOOP ( 'NONE', ( #39109, #2326, #14048, #42847 ) ) ;
#6730=DIRECTION ( 'NONE',  ( 1.000000000000000000, -0.000000000000000000, -0.000000000000000000 ) ) ;
#6738=DIRECTION ( 'NONE',  ( 0.000000000000000000, 0.000000000000000000, 1.000000000000000000 ) ) ;
#6751=DIRECTION ( 'NONE',  ( 0.000000000000000000, 0.000000000000000000, 1.000000000000000000 ) ) ;
#6768=ORIENTED_EDGE ( 'NONE', *, *, #42448, .T. ) ;
#6774=CARTESIAN_POINT ( 'NONE',  ( 784.4999999999993179, -513.1383975375929367, -367.9999999999999432 ) ) ;
#6778=DIRECTION ( 'NONE',  ( 1.000000000000000000, 0.000000000000000000, 0.000000000000000000 ) ) ;
#6787=DIRECTION ( 'NONE',  ( -1.000000000000000000, -0.000000000000000000, -0.000000000000000000 ) ) ;
#6800=DIRECTION ( 'NONE',  ( 1.000000000000000000, 0.000000000000000000, -0.000000000000000000 ) ) ;
#6828=DIRECTION ( 'NONE',  ( -0.000000000000000000, -0.3826834323650838421, -0.9238795325112891810 ) ) ;
#6862=EDGE_CURVE ( 'NONE', #42371, #40010, #8571, .T. ) ;
#6878=AXIS2_PLACEMENT_3D ( 'NONE', #2955, #24878, #31803 ) ;
#6898=ORIENTED_EDGE ( 'NONE', *, *, #29198, .T. ) ;
#6902=VECTOR ( 'NONE', #40429, 1000.000000000000000 ) ;
#6908=EDGE_CURVE ( 'NONE', #1390, #6318, #25029, .T. ) ;
#6951=VECTOR ( 'NONE', #34287, 1000.000000000000000 ) ;
#6954=EDGE_LOOP ( 'NONE', ( #33679, #29390, #23621, #12123 ) ) ;
#6964=EDGE_CURVE ( 'NONE', #24418, #16954, #29854, .T. ) ;
#6987=DIRECTION ( 'NONE',  ( 0.000000000000000000, -0.9238795325112892920, 0.3826834323650836756 ) ) ;
#6998=DIRECTION ( 'NONE',  ( 0.000000000000000000, 0.6755902076156505842, 0.7372773368101327440 ) ) ;
#7004=CLOSED_SHELL ( 'NONE', ( #11735, #8851, #8351, #2085, #35382, #6276, #36538, #13914 ) ) ;
#7024=DIRECTION ( 'NONE',  ( -1.000000000000000000, -0.000000000000000000, 0.000000000000000000 ) ) ;
#7025=DIRECTION ( 'NONE',  ( -1.000000000000000000, -0.000000000000000000, -0.000000000000000000 ) ) ;
#7048=CARTESIAN_POINT ( 'NONE',  ( -28.63011601220122415, -496.5085659523897448, -356.8883017825714319 ) ) ;
#7058=ORIENTED_EDGE ( 'NONE', *, *, #17396, .F. ) ;
#7060=VECTOR ( 'NONE', #39739, 1000.000000000000114 ) ;
#7077=ORIENTED_EDGE ( 'NONE', *, *, #16579, .T. ) ;
#7102=CARTESIAN_POINT ( 'NONE',  ( -784.4999999999993179, -365.3551492539851893, -18.13243251470705886 ) ) ;
#7103=CARTESIAN_POINT ( 'NONE',  ( 786.4999999999993179, -110.5936016518799221, 750.6326042729449455 ) ) ;
#7110=CARTESIAN_POINT ( 'NONE',  ( 786.4999999999993179, 22.32581219114657856, 895.6886905569881492 ) ) ;
#7122=ORIENTED_EDGE ( 'NONE', *, *, #26985, .F. ) ;
#7141=DIRECTION ( 'NONE',  ( 1.000000000000000000, -0.000000000000000000, -0.000000000000000000 ) ) ;
#7148=EDGE_CURVE ( 'NONE', #40010, #30797, #8630, .T. ) ;
#7155=VECTOR ( 'NONE', #7141, 1000.000000000000000 ) ;
#7158=VECTOR ( 'NONE', #1763, 1000.000000000000000 ) ;
#7163=DIRECTION ( 'NONE',  ( 0.000000000000000000, 0.000000000000000000, 1.000000000000000000 ) ) ;
#7214=ADVANCED_FACE ( 'NONE', ( #26604 ), #44167, .T. ) ;
#7217=DIRECTION ( 'NONE',  ( -1.000000000000000000, -0.000000000000000000, -0.000000000000000000 ) ) ;
#7229=CIRCLE ( 'NONE', #2056, 18.00000000000001421 ) ;
#7243=EDGE_CURVE ( 'NONE', #1813, #2103, #19916, .T. ) ;
#7248=ORIENTED_EDGE ( 'NONE', *, *, #15570, .F. ) ;
#7251=ORIENTED_EDGE ( 'NONE', *, *, #5182, .T. ) ;
#7259=CARTESIAN_POINT ( 'NONE',  ( -775.4999999999993179, -512.9681489794448908, -339.9999999999999432 ) ) ;
#7264=VECTOR ( 'NONE', #7403, 1000.000000000000000 ) ;
#7274=CARTESIAN_POINT ( 'NONE',  ( 786.4999999999993179, -512.9681489794448908, -339.9999999999999432 ) ) ;
#7353=ORIENTED_EDGE ( 'NONE', *, *, #15376, .F. ) ;
#7364=DIRECTION ( 'NONE',  ( 0.000000000000000000, -0.9238795325112892920, 0.3826834323650836756 ) ) ;
#7369=DIRECTION ( 'NONE',  ( -1.000000000000000000, -0.000000000000000000, -0.000000000000000000 ) ) ;
#7382=DIRECTION ( 'NONE',  ( 0.000000000000000000, -0.6755902076156505842, -0.7372773368101328550 ) ) ;
#7393=ADVANCED_FACE ( 'NONE', ( #41172, #44627 ), #44391, .F. ) ;
#7403=DIRECTION ( 'NONE',  ( 0.000000000000000000, 0.000000000000000000, -1.000000000000000000 ) ) ;
#7404=VERTEX_POINT ( 'NONE', #5831 ) ;
#7440=EDGE_CURVE ( 'NONE', #23506, #11791, #29629, .T. ) ;
#7478=VERTEX_POINT ( 'NONE', #31452 ) ;
#7481=CARTESIAN_POINT ( 'NONE',  ( -786.4999999999993179, -544.8427095258973623, -350.0000000000000000 ) ) ;
#7514=DIRECTION ( 'NONE',  ( -1.000000000000000000, -0.000000000000000000, -0.000000000000000000 ) ) ;
#7543=DIRECTION ( 'NONE',  ( 0.000000000000000000, 0.000000000000000000, 1.000000000000000000 ) ) ;
#7562=DIRECTION ( 'NONE',  ( 0.000000000000000000, 0.000000000000000000, 1.000000000000000000 ) ) ;
#7564=ORIENTED_EDGE ( 'NONE', *, *, #41585, .F. ) ;
#7593=LINE ( 'NONE', #27687, #18246 ) ;
#7685=VECTOR ( 'NONE', #1888, 1000.000000000000114 ) ;
#7686=ORIENTED_EDGE ( 'NONE', *, *, #11685, .F. ) ;
#7708=DIRECTION ( 'NONE',  ( -0.000000000000000000, -0.6755902076156505842, -0.7372773368101328550 ) ) ;
#7710=CARTESIAN_POINT ( 'NONE',  ( 786.4999999999993179, -513.1383975375929367, -369.9999999999999432 ) ) ;
#7713=DIRECTION ( 'NONE',  ( -1.000000000000000000, -0.000000000000000000, 0.000000000000000000 ) ) ;
#7728=FACE_OUTER_BOUND ( 'NONE', #22615, .T. ) ;
#7757=CIRCLE ( 'NONE', #23219, 12.00000000000001066 ) ;
#7768=PLANE ( 'NONE',  #43890 ) ;
#7779=DIRECTION ( 'NONE',  ( 0.000000000000000000, 0.000000000000000000, 1.000000000000000000 ) ) ;
#7786=DIRECTION ( 'NONE',  ( -1.000000000000000000, 0.000000000000000000, 0.000000000000000000 ) ) ;
#7795=DIRECTION ( 'NONE',  ( 0.000000000000000000, 0.3826834323650838421, 0.9238795325112891810 ) ) ;
#7798=ORIENTED_EDGE ( 'NONE', *, *, #21358, .T. ) ;
#7806=VERTEX_POINT ( 'NONE', #22191 ) ;
#7809=CIRCLE ( 'NONE', #20960, 12.00000000000001066 ) ;
#7810=EDGE_CURVE ( 'NONE', #30700, #40621, #36511, .T. ) ;
#7813=CIRCLE ( 'NONE', #17399, 18.00000000000001421 ) ;
#7814=VERTEX_POINT ( 'NONE', #32825 ) ;
#7826=DIRECTION ( 'NONE',  ( 0.000000000000000000, 0.000000000000000000, -1.000000000000000000 ) ) ;
#7836=LINE ( 'NONE', #42467, #12729 ) ;
#7844=DIRECTION ( 'NONE',  ( 1.000000000000000000, 0.000000000000000000, -0.000000000000000000 ) ) ;
#7856=VERTEX_POINT ( 'NONE', #501 ) ;
#7882=ORIENTED_EDGE ( 'NONE', *, *, #41294, .F. ) ;
#7924=VECTOR ( 'NONE', #31830, 1000.000000000000114 ) ;
#7954=PLANE ( 'NONE',  #42983 ) ;
#7979=UNCERTAINTY_MEASURE_WITH_UNIT (LENGTH_MEASURE( 1.000000000000000082E-05 ), #38802, 'distance_accuracy_value', 'NONE');
#7981=DIRECTION ( 'NONE',  ( 0.000000000000000000, 0.000000000000000000, 1.000000000000000000 ) ) ;
#7983=EDGE_CURVE ( 'NONE', #7806, #37281, #12188, .T. ) ;
#7984=VERTEX_POINT ( 'NONE', #25879 ) ;
#8010=LINE ( 'NONE', #21849, #37035 ) ;
#8011=FACE_BOUND ( 'NONE', #12913, .T. ) ;
#8044=ORIENTED_EDGE ( 'NONE', *, *, #41026, .T. ) ;
#8066=DIRECTION ( 'NONE',  ( 1.000000000000000000, -0.000000000000000000, -0.000000000000000000 ) ) ;
#8098=DIRECTION ( 'NONE',  ( 1.000000000000000000, -0.000000000000000000, -0.000000000000000000 ) ) ;
#8099=ORIENTED_EDGE ( 'NONE', *, *, #42697, .T. ) ;
#8107=EDGE_LOOP ( 'NONE', ( #36094, #15933 ) ) ;
#8124=CARTESIAN_POINT ( 'NONE',  ( -786.4999999999993179, -513.1383975375929367, -369.9999999999999432 ) ) ;
#8194=CARTESIAN_POINT ( 'NONE',  ( -773.4999999999993179, -365.3551492539851893, -18.13243251470705886 ) ) ;
#8222=CARTESIAN_POINT ( 'NONE',  ( 773.4999999999993179, -544.8427095258973623, -350.0000000000000000 ) ) ;
#8238=DIRECTION ( 'NONE',  ( 0.000000000000000000, 0.9238795325112891810, -0.3826834323650838421 ) ) ;
#8243=VECTOR ( 'NONE', #36501, 1000.000000000000227 ) ;
#8253=ORIENTED_EDGE ( 'NONE', *, *, #31216, .F. ) ;
#8270=CARTESIAN_POINT ( 'NONE',  ( 786.4999999999993179, 26.27639943461401018, 900.0000000000001137 ) ) ;
#8319=EDGE_CURVE ( 'NONE', #3612, #41109, #45393, .T. ) ;
#8320=CARTESIAN_POINT ( 'NONE',  ( 784.4999999999993179, -563.3203001761231690, -342.3463313526983143 ) ) ;
#8343=DIRECTION ( 'NONE',  ( 0.000000000000000000, 0.000000000000000000, 1.000000000000000000 ) ) ;
#8351=ADVANCED_FACE ( 'NONE', ( #2529 ), #13173, .F. ) ;
#8360=DIRECTION ( 'NONE',  ( -1.000000000000000000, -0.000000000000000000, -0.000000000000000000 ) ) ;
#8379=CARTESIAN_POINT ( 'NONE',  ( -775.4999999999993179, -512.9681489794448908, -327.9999999999999432 ) ) ;
#8418=ORIENTED_EDGE ( 'NONE', *, *, #38068, .T. ) ;
#8457=LINE ( 'NONE', #22761, #43829 ) ;
#8477=CIRCLE ( 'NONE', #20263, 9.999999999999982236 ) ;
#8480=AXIS2_PLACEMENT_3D ( 'NONE', #5426, #19300, #15612 ) ;
#8493=VECTOR ( 'NONE', #20143, 999.9999999999998863 ) ;
#8516=AXIS2_PLACEMENT_3D ( 'NONE', #36131, #25731, #28267 ) ;
#8555=ORIENTED_EDGE ( 'NONE', *, *, #18304, .F. ) ;
#8559=FACE_OUTER_BOUND ( 'NONE', #13422, .T. ) ;
#8571=CIRCLE ( 'NONE', #15834, 9.999999999999982236 ) ;
#8574=AXIS2_PLACEMENT_3D ( 'NONE', #11453, #25536, #42643 ) ;
#8580=CARTESIAN_POINT ( 'NONE',  ( -786.4999999999993179, -513.1383975375929367, -349.9999999999999432 ) ) ;
#8597=CARTESIAN_POINT ( 'NONE',  ( 1007.605605532488426, -434.0043448692482002, 397.6917108626901154 ) ) ;
#8604=EDGE_CURVE ( 'NONE', #17065, #23212, #29206, .T. ) ;
#8630=LINE ( 'NONE', #19232, #4047 ) ;
#8639=ORIENTED_EDGE ( 'NONE', *, *, #32957, .T. ) ;
#8654=CARTESIAN_POINT ( 'NONE',  ( -26.63011601220122060, -512.9681489794448908, -329.9999999999999432 ) ) ;
#8660=EDGE_CURVE ( 'NONE', #1029, #5066, #44036, .T. ) ;
#8672=DIRECTION ( 'NONE',  ( 0.000000000000000000, 0.000000000000000000, 1.000000000000000000 ) ) ;
#8690=DIRECTION ( 'NONE',  ( 0.000000000000000000, -0.6755902076156505842, -0.7372773368101327440 ) ) ;
#8697=DIRECTION ( 'NONE',  ( 1.000000000000000000, -0.000000000000000000, -0.000000000000000000 ) ) ;
#8718=ORIENTED_EDGE ( 'NONE', *, *, #30332, .F. ) ;
#8720=ORIENTED_EDGE ( 'NONE', *, *, #7243, .F. ) ;
#8726=DIRECTION ( 'NONE',  ( 0.000000000000000000, -0.3826834323650835645, -0.9238795325112892920 ) ) ;
#8734=LINE ( 'NONE', #16326, #27061 ) ;
#8747=VERTEX_POINT ( 'NONE', #40128 ) ;
#8784=ORIENTED_EDGE ( 'NONE', *, *, #26936, .T. ) ;
#8798=VECTOR ( 'NONE', #43446, 1000.000000000000000 ) ;
#8801=ADVANCED_FACE ( 'NONE', ( #26262 ), #36666, .F. ) ;
#8824=ORIENTED_EDGE ( 'NONE', *, *, #6060, .T. ) ;
#8844=DIRECTION ( 'NONE',  ( 1.000000000000000000, -0.000000000000000000, -0.000000000000000000 ) ) ;
#8851=ADVANCED_FACE ( 'NONE', ( #29720 ), #43798, .F. ) ;
#8894=LINE ( 'NONE', #6101, #17187 ) ;
#8899=DIRECTION ( 'NONE',  ( 0.000000000000000000, 0.000000000000000000, 1.000000000000000000 ) ) ;
#8933=DIRECTION ( 'NONE',  ( 1.000000000000000000, -0.000000000000000000, -0.000000000000000000 ) ) ;
#8951=ORIENTED_EDGE ( 'NONE', *, *, #22178, .F. ) ;
#8954=CARTESIAN_POINT ( 'NONE',  ( -39.63011601220123481, -494.6608068873671300, -357.6536686473015720 ) ) ;
#8957=DIRECTION ( 'NONE',  ( 1.000000000000000000, -0.000000000000000000, -0.000000000000000000 ) ) ;
#8969=CARTESIAN_POINT ( 'NONE',  ( 786.4999999999993179, -513.1383975375929367, -369.9999999999999432 ) ) ;
#8994=CYLINDRICAL_SURFACE ( 'NONE', #14301, 9.999999999999980460 ) ;
#9053=DIRECTION ( 'NONE',  ( 1.000000000000000000, 0.000000000000000000, 0.000000000000000000 ) ) ;
#9060=DIRECTION ( 'NONE',  ( 0.000000000000000000, -0.3826834323650836756, -0.9238795325112892920 ) ) ;
#9075=LINE ( 'NONE', #37246, #19600 ) ;
#9077=ORIENTED_EDGE ( 'NONE', *, *, #7983, .F. ) ;
#9097=EDGE_CURVE ( 'NONE', #14962, #40161, #38263, .T. ) ;
#9103=ORIENTED_EDGE ( 'NONE', *, *, #4891, .F. ) ;
#9110=FACE_OUTER_BOUND ( 'NONE', #12110, .T. ) ;
#9112=LINE ( 'NONE', #29678, #11966 ) ;
#9117=CARTESIAN_POINT ( 'NONE',  ( 773.4999999999993179, -512.9681489794448908, -339.9999999999999432 ) ) ;
#9120=DIRECTION ( 'NONE',  ( -1.000000000000000000, -0.000000000000000000, -0.000000000000000000 ) ) ;
#9121=CARTESIAN_POINT ( 'NONE',  ( -786.4999999999993179, -110.5936016518799221, 750.6326042729449455 ) ) ;
#9123=AXIS2_PLACEMENT_3D ( 'NONE', #33107, #15329, #37224 ) ;
#9142=CARTESIAN_POINT ( 'NONE',  ( -786.4999999999993179, -513.1383975375929367, -369.9999999999999432 ) ) ;
#9159=CARTESIAN_POINT ( 'NONE',  ( 786.4999999999993179, 26.27639943461401018, 900.0000000000001137 ) ) ;
#9169=CARTESIAN_POINT ( 'NONE',  ( 786.4999999999993179, -563.3203001761230553, -342.3463313526983143 ) ) ;
#9196=VECTOR ( 'NONE', #32491, 1000.000000000000227 ) ;
#9232=VECTOR ( 'NONE', #8957, 1000.000000000000000 ) ;
#9251=AXIS2_PLACEMENT_3D ( 'NONE', #9159, #1755, #19116 ) ;
#9279=VERTEX_POINT ( 'NONE', #31992 ) ;
#9315=VERTEX_POINT ( 'NONE', #11681 ) ;
#9336=DIRECTION ( 'NONE',  ( -1.000000000000000000, -0.000000000000000000, -0.000000000000000000 ) ) ;
#9339=ORIENTED_EDGE ( 'NONE', *, *, #23300, .F. ) ;
#9360=DIRECTION ( 'NONE',  ( -0.000000000000000000, 1.000000000000000000, -0.000000000000000000 ) ) ;
#9362=VECTOR ( 'NONE', #44617, 1000.000000000000227 ) ;
#9367=CIRCLE ( 'NONE', #35174, 10.00000000000000888 ) ;
#9386=VECTOR ( 'NONE', #26715, 1000.000000000000114 ) ;
#9404=CARTESIAN_POINT ( 'NONE',  ( 1007.605605532488426, -436.2161768796786987, 399.7184814855371542 ) ) ;
#9410=ORIENTED_EDGE ( 'NONE', *, *, #34612, .T. ) ;
#9416=EDGE_CURVE ( 'NONE', #601, #25954, #7813, .T. ) ;
#9433=LINE ( 'NONE', #2257, #1923 ) ;
#9436=EDGE_LOOP ( 'NONE', ( #23360, #45651, #40241, #764, #33427, #15880 ) ) ;
#9454=ORIENTED_EDGE ( 'NONE', *, *, #8319, .F. ) ;
#9455=CIRCLE ( 'NONE', #35267, 10.00000000000000888 ) ;
#9550=CARTESIAN_POINT ( 'NONE',  ( -786.4999999999993179, 26.27639943461401018, 900.0000000000001137 ) ) ;
#9585=DIRECTION ( 'NONE',  ( -1.000000000000000000, -0.000000000000000000, -0.000000000000000000 ) ) ;
#9652=ORIENTED_EDGE ( 'NONE', *, *, #11738, .T. ) ;
#9669=EDGE_CURVE ( 'NONE', #11791, #10012, #33638, .T. ) ;
#9698=ADVANCED_FACE ( 'NONE', ( #44209 ), #26644, .F. ) ;
#9710=ORIENTED_EDGE ( 'NONE', *, *, #9416, .T. ) ;
#9721=ADVANCED_FACE ( 'NONE', ( #12569 ), #12785, .F. ) ;
#9741=CARTESIAN_POINT ( 'NONE',  ( -26.63011601220122060, -544.8427095258973623, -369.9999999999999432 ) ) ;
#9745=CARTESIAN_POINT ( 'NONE',  ( 773.4999999999993179, -513.1383975375929367, -369.9999999999999432 ) ) ;
#9768=VECTOR ( 'NONE', #45196, 1000.000000000000000 ) ;
#9780=EDGE_LOOP ( 'NONE', ( #37451, #20911, #29168, #1816 ) ) ;
#9784=EDGE_CURVE ( 'NONE', #39697, #36781, #33816, .T. ) ;
#9788=ORIENTED_EDGE ( 'NONE', *, *, #41294, .T. ) ;
#9807=CARTESIAN_POINT ( 'NONE',  ( -26.63011601220122060, -513.1383975375929367, -349.9999999999999432 ) ) ;
#9836=AXIS2_PLACEMENT_3D ( 'NONE', #21729, #45612, #39774 ) ;
#9867=EDGE_LOOP ( 'NONE', ( #18095, #26764, #8253, #12212, #34371, #25364 ) ) ;
#9897=CIRCLE ( 'NONE', #43884, 10.00000000000000888 ) ;
#9904=DIRECTION ( 'NONE',  ( -1.000000000000000000, -0.000000000000000000, -0.000000000000000000 ) ) ;
#9977=AXIS2_PLACEMENT_3D ( 'NONE', #28805, #8238, #7795 ) ;
#10002=AXIS2_PLACEMENT_3D ( 'NONE', #30261, #33740, #37885 ) ;
#10012=VERTEX_POINT ( 'NONE', #17172 ) ;
#10019=ADVANCED_FACE ( 'NONE', ( #24319 ), #27560, .T. ) ;
#10023=AXIS2_PLACEMENT_3D ( 'NONE', #25756, #28294, #42853 ) ;
#10029=ORIENTED_EDGE ( 'NONE', *, *, #40804, .F. ) ;
#10056=LINE ( 'NONE', #31289, #26171 ) ;
#10066=CARTESIAN_POINT ( 'NONE',  ( -784.4999999999993179, -365.3551492539851893, -18.13243251470705886 ) ) ;
#10099=EDGE_CURVE ( 'NONE', #17152, #32355, #20176, .T. ) ;
#10103=LINE ( 'NONE', #27417, #44866 ) ;
#10121=AXIS2_PLACEMENT_3D ( 'NONE', #25301, #39412, #21843 ) ;
#10137=ORIENTED_EDGE ( 'NONE', *, *, #15665, .T. ) ;
#10145=ORIENTED_EDGE ( 'NONE', *, *, #21098, .F. ) ;
#10176=ORIENTED_EDGE ( 'NONE', *, *, #25485, .F. ) ;
#10186=ORIENTED_EDGE ( 'NONE', *, *, #24165, .F. ) ;
#10193=FACE_BOUND ( 'NONE', #19044, .T. ) ;
#10232=ORIENTED_EDGE ( 'NONE', *, *, #25795, .F. ) ;
#10236=AXIS2_PLACEMENT_3D ( 'NONE', #17139, #7217, #24505 ) ;
#10285=VERTEX_POINT ( 'NONE', #6774 ) ;
#10307=VECTOR ( 'NONE', #13946, 1000.000000000000114 ) ;
#10320=DIRECTION ( 'NONE',  ( 0.000000000000000000, 0.000000000000000000, 1.000000000000000000 ) ) ;
#10339=VERTEX_POINT ( 'NONE', #17864 ) ;
#10346=ADVANCED_FACE ( 'NONE', ( #18100 ), #14405, .F. ) ;
#10416=CARTESIAN_POINT ( 'NONE',  ( -28.63011601220122415, -544.8427095258973623, -350.0000000000000000 ) ) ;
#10451=FACE_OUTER_BOUND ( 'NONE', #24773, .T. ) ;
#10466=EDGE_LOOP ( 'NONE', ( #2897, #28930, #10623, #28009 ) ) ;
#10469=DIRECTION ( 'NONE',  ( 0.000000000000000000, 0.000000000000000000, 1.000000000000000000 ) ) ;
#10470=ORIENTED_EDGE ( 'NONE', *, *, #21358, .F. ) ;
#10478=DIRECTION ( 'NONE',  ( -1.000000000000000000, -0.000000000000000000, 0.000000000000000000 ) ) ;
#10484=DIRECTION ( 'NONE',  ( 0.000000000000000000, 0.000000000000000000, 1.000000000000000000 ) ) ;
#10496=LINE ( 'NONE', #13980, #14421 ) ;
#10500=ORIENTED_EDGE ( 'NONE', *, *, #21278, .T. ) ;
#10520=FACE_BOUND ( 'NONE', #11836, .T. ) ;
#10526=AXIS2_PLACEMENT_3D ( 'NONE', #8222, #22291, #32943 ) ;
#10544=DIRECTION ( 'NONE',  ( -1.000000000000000000, 0.000000000000000000, 0.000000000000000000 ) ) ;
#10563=ORIENTED_EDGE ( 'NONE', *, *, #7440, .T. ) ;
#10569=EDGE_LOOP ( 'NONE', ( #2212, #17051, #4271, #3809 ) ) ;
#10584=EDGE_CURVE ( 'NONE', #518, #38954, #6385, .T. ) ;
#10588=DIRECTION ( 'NONE',  ( 1.000000000000000000, -0.000000000000000000, -0.000000000000000000 ) ) ;
#10598=AXIS2_PLACEMENT_3D ( 'NONE', #22183, #7025, #28033 ) ;
#10609=EDGE_CURVE ( 'NONE', #14297, #16495, #39344, .T. ) ;
#10623=ORIENTED_EDGE ( 'NONE', *, *, #40528, .T. ) ;
#10630=EDGE_LOOP ( 'NONE', ( #39870, #1360, #22832, #19224 ) ) ;
#10659=DIRECTION ( 'NONE',  ( -1.000000000000000000, -0.000000000000000000, 0.000000000000000000 ) ) ;
#10664=CYLINDRICAL_SURFACE ( 'NONE', #10236, 12.00000000000001066 ) ;
#10686=DIRECTION ( 'NONE',  ( 1.000000000000000000, 0.000000000000000000, 0.000000000000000000 ) ) ;
#10702=DIRECTION ( 'NONE',  ( 1.000000000000000000, -0.000000000000000000, -0.000000000000000000 ) ) ;
#10718=AXIS2_PLACEMENT_3D ( 'NONE', #10416, #3263, #40751 ) ;
#10723=CARTESIAN_POINT ( 'NONE',  ( -26.63011601220122060, -512.9681489794448908, -350.0000000000000000 ) ) ;
#10736=CARTESIAN_POINT ( 'NONE',  ( -786.4999999999993179, -513.1383975375929367, -349.9999999999999432 ) ) ;
#10763=DIRECTION ( 'NONE',  ( 1.000000000000000000, 0.000000000000000000, 0.000000000000000000 ) ) ;
#10784=CYLINDRICAL_SURFACE ( 'NONE', #14299, 12.00000000000001066 ) ;
#10794=DIRECTION ( 'NONE',  ( 0.000000000000000000, 0.000000000000000000, 1.000000000000000000 ) ) ;
#10827=FACE_BOUND ( 'NONE', #2163, .T. ) ;
#10832=LINE ( 'NONE', #38542, #7155 ) ;
#10845=EDGE_CURVE ( 'NONE', #1374, #34451, #44728, .T. ) ;
#10873=EDGE_LOOP ( 'NONE', ( #694, #12394, #3705, #1320 ) ) ;
#10885=PLANE ( 'NONE',  #40307 ) ;
#10906=DIRECTION ( 'NONE',  ( 0.000000000000000000, 0.000000000000000000, -1.000000000000000000 ) ) ;
#10954=CARTESIAN_POINT ( 'NONE',  ( -773.4999999999993179, -544.8427095258973623, -369.9999999999999432 ) ) ;
#10993=ORIENTED_EDGE ( 'NONE', *, *, #31782, .T. ) ;
#10999=PLANE ( 'NONE',  #26242 ) ;
#11013=DIRECTION ( 'NONE',  ( 1.000000000000000000, 0.000000000000000000, -0.000000000000000000 ) ) ;
#11037=ORIENTED_EDGE ( 'NONE', *, *, #20142, .F. ) ;
#11108=ORIENTED_EDGE ( 'NONE', *, *, #23827, .F. ) ;
#11172=CARTESIAN_POINT ( 'NONE',  ( -28.63011601220122415, -501.1515549466498669, -368.0974687824633520 ) ) ;
#11216=ORIENTED_EDGE ( 'NONE', *, *, #24165, .T. ) ;
#11223=VERTEX_POINT ( 'NONE', #35299 ) ;
#11245=CARTESIAN_POINT ( 'NONE',  ( -775.4999999999993179, -355.4967352946684969, -16.45562775363632113 ) ) ;
#11264=ORIENTED_EDGE ( 'NONE', *, *, #988, .F. ) ;
#11276=CYLINDRICAL_SURFACE ( 'NONE', #18434, 9.999999999999980460 ) ;
#11281=DIRECTION ( 'NONE',  ( -1.000000000000000000, -0.000000000000000000, 0.000000000000000000 ) ) ;
#11283=CARTESIAN_POINT ( 'NONE',  ( -28.63011601220122415, -513.1383975375929367, -369.9999999999999432 ) ) ;
#11297=DIRECTION ( 'NONE',  ( 0.000000000000000000, 0.000000000000000000, 1.000000000000000000 ) ) ;
#11318=LINE ( 'NONE', #25162, #7264 ) ;
#11352=CARTESIAN_POINT ( 'NONE',  ( -775.4999999999993179, -544.8427095258973623, -350.0000000000000000 ) ) ;
#11375=ORIENTED_EDGE ( 'NONE', *, *, #6060, .F. ) ;
#11379=ORIENTED_EDGE ( 'NONE', *, *, #27521, .T. ) ;
#11394=CIRCLE ( 'NONE', #25396, 9.999999999999982236 ) ;
#11401=CARTESIAN_POINT ( 'NONE',  ( 746.4999999999993179, -365.3551492539851893, -28.13243251470704109 ) ) ;
#11427=CARTESIAN_POINT ( 'NONE',  ( 786.4999999999993179, -544.8427095258973623, -350.0000000000000000 ) ) ;
#11429=EDGE_CURVE ( 'NONE', #35816, #22547, #43380, .T. ) ;
#11432=VECTOR ( 'NONE', #12992, 1000.000000000000000 ) ;
#11438=ORIENTED_EDGE ( 'NONE', *, *, #21258, .T. ) ;
#11453=CARTESIAN_POINT ( 'NONE',  ( 746.4999999999993179, -365.3551492539851893, -18.13243251470705886 ) ) ;
#11458=EDGE_CURVE ( 'NONE', #31246, #35031, #18905, .T. ) ;
#11470=CYLINDRICAL_SURFACE ( 'NONE', #2475, 19.99999999999990763 ) ;
#11477=EDGE_CURVE ( 'NONE', #33295, #44478, #39713, .T. ) ;
#11478=DIRECTION ( 'NONE',  ( 0.000000000000000000, 0.000000000000000000, -1.000000000000000000 ) ) ;
#11481=AXIS2_PLACEMENT_3D ( 'NONE', #15941, #44337, #12692 ) ;
#11488=ORIENTED_EDGE ( 'NONE', *, *, #6611, .F. ) ;
#11499=ORIENTED_EDGE ( 'NONE', *, *, #32094, .F. ) ;
#11511=DIRECTION ( 'NONE',  ( -0.000000000000000000, -0.3826834323650836756, -0.9238795325112892920 ) ) ;
#11519=EDGE_CURVE ( 'NONE', #40621, #22833, #32207, .T. ) ;
#11535=LINE ( 'NONE', #39033, #42442 ) ;
#11540=DIRECTION ( 'NONE',  ( 0.000000000000000000, 0.000000000000000000, 1.000000000000000000 ) ) ;
#11546=PLANE ( 'NONE',  #38780 ) ;
#11555=LINE ( 'NONE', #4397, #17301 ) ;
#11570=CIRCLE ( 'NONE', #43278, 9.999999999999980460 ) ;
#11592=DIRECTION ( 'NONE',  ( 1.000000000000000000, -0.000000000000000000, -0.000000000000000000 ) ) ;
#11595=CARTESIAN_POINT ( 'NONE',  ( 786.4999999999993179, -112.8054336623104348, 752.6593748957919843 ) ) ;
#11606=VECTOR ( 'NONE', #19338, 1000.000000000000114 ) ;
#11655=DIRECTION ( 'NONE',  ( 0.000000000000000000, 0.7372773368101421809, -0.6755902076156404812 ) ) ;
#11656=DIRECTION ( 'NONE',  ( 0.000000000000000000, 0.000000000000000000, 1.000000000000000000 ) ) ;
#11663=FACE_OUTER_BOUND ( 'NONE', #18420, .T. ) ;
#11680=DIRECTION ( 'NONE',  ( 1.000000000000000000, 0.000000000000000000, -0.000000000000000000 ) ) ;
#11681=CARTESIAN_POINT ( 'NONE',  ( 786.4999999999993179, -512.9681489794448908, -329.9999999999999432 ) ) ;
#11685=EDGE_CURVE ( 'NONE', #23212, #32281, #41044, .T. ) ;
#11687=DIRECTION ( 'NONE',  ( 1.000000000000000000, -0.000000000000000000, -0.000000000000000000 ) ) ;
#11695=CARTESIAN_POINT ( 'NONE',  ( -746.4999999999993179, -365.3551492539851893, -8.132432514707076621 ) ) ;
#11715=EDGE_LOOP ( 'NONE', ( #1556, #13243, #8639, #15571 ) ) ;
#11735=ADVANCED_FACE ( 'NONE', ( #5708 ), #19559, .F. ) ;
#11738=EDGE_CURVE ( 'NONE', #40310, #29646, #2731, .T. ) ;
#11742=FACE_OUTER_BOUND ( 'NONE', #22058, .T. ) ;
#11744=LINE ( 'NONE', #36434, #40254 ) ;
#11748=DIRECTION ( 'NONE',  ( -1.000000000000000000, 0.000000000000000000, 0.000000000000000000 ) ) ;
#11772=CARTESIAN_POINT ( 'NONE',  ( 775.4999999999993179, -857.0166862835568509, -63.94525337997358605 ) ) ;
#11791=VERTEX_POINT ( 'NONE', #2460 ) ;
#11836=EDGE_LOOP ( 'NONE', ( #34716, #2943 ) ) ;
#11840=VERTEX_POINT ( 'NONE', #26945 ) ;
#11847=CARTESIAN_POINT ( 'NONE',  ( -773.4999999999993179, -512.9681489794448908, -329.9999999999999432 ) ) ;
#11851=DIRECTION ( 'NONE',  ( 0.000000000000000000, 0.000000000000000000, 1.000000000000000000 ) ) ;
#11853=PLANE ( 'NONE',  #17166 ) ;
#11876=EDGE_CURVE ( 'NONE', #19577, #3612, #8734, .T. ) ;
#11895=EDGE_CURVE ( 'NONE', #38954, #14962, #23012, .T. ) ;
#11926=EDGE_CURVE ( 'NONE', #40161, #44892, #22800, .T. ) ;
#11958=CARTESIAN_POINT ( 'NONE',  ( -773.4999999999993179, -544.8427095258973623, -350.0000000000000000 ) ) ;
#11966=VECTOR ( 'NONE', #12368, 1000.000000000000114 ) ;
#11969=LINE ( 'NONE', #1114, #32270 ) ;
#11992=ORIENTED_EDGE ( 'NONE', *, *, #35171, .F. ) ;
#12035=LINE ( 'NONE', #26103, #4041 ) ;
#12065=ORIENTED_EDGE ( 'NONE', *, *, #17608, .T. ) ;
#12077=DIRECTION ( 'NONE',  ( 0.000000000000000000, -0.9238795325112892920, 0.3826834323650836756 ) ) ;
#12087=DIRECTION ( 'NONE',  ( 0.000000000000000000, -0.9238795325112892920, 0.3826834323650836756 ) ) ;
#12110=EDGE_LOOP ( 'NONE', ( #44312, #2847, #235, #25524 ) ) ;
#12123=ORIENTED_EDGE ( 'NONE', *, *, #19325, .T. ) ;
#12125=CARTESIAN_POINT ( 'NONE',  ( 786.4999999999993179, -513.1383975375929367, -369.9999999999999432 ) ) ;
#12141=LINE ( 'NONE', #19751, #37895 ) ;
#12156=CARTESIAN_POINT ( 'NONE',  ( 775.4999999999993179, -365.3551492539851893, -8.132432514707076621 ) ) ;
#12179=CARTESIAN_POINT ( 'NONE',  ( 1007.605605532488426, -292.9981031064102126, 121.3637880562633171 ) ) ;
#12188=CIRCLE ( 'NONE', #1103, 12.00000000000001066 ) ;
#12212=ORIENTED_EDGE ( 'NONE', *, *, #30317, .T. ) ;
#12245=EDGE_CURVE ( 'NONE', #41109, #23212, #41500, .T. ) ;
#12302=ADVANCED_FACE ( 'NONE', ( #32248 ), #36382, .F. ) ;
#12341=ORIENTED_EDGE ( 'NONE', *, *, #38798, .F. ) ;
#12368=DIRECTION ( 'NONE',  ( -0.000000000000000000, 0.6755902076156502511, 0.7372773368101330771 ) ) ;
#12394=ORIENTED_EDGE ( 'NONE', *, *, #11458, .F. ) ;
#12423=VECTOR ( 'NONE', #42662, 1000.000000000000000 ) ;
#12482=LINE ( 'NONE', #16172, #39046 ) ;
#12490=CYLINDRICAL_SURFACE ( 'NONE', #34328, 10.00000000000000888 ) ;
#12516=EDGE_CURVE ( 'NONE', #36107, #25758, #25302, .T. ) ;
#12530=DIRECTION ( 'NONE',  ( -1.000000000000000000, -0.000000000000000000, -0.000000000000000000 ) ) ;
#12553=CARTESIAN_POINT ( 'NONE',  ( -786.4999999999993179, -513.1383975375929367, -369.9999999999999432 ) ) ;
#12557=CARTESIAN_POINT ( 'NONE',  ( 775.4999999999993179, -512.9681489794448908, -352.0000000000000000 ) ) ;
#12569=FACE_OUTER_BOUND ( 'NONE', #14340, .T. ) ;
#12619=ORIENTED_EDGE ( 'NONE', *, *, #22408, .F. ) ;
#12636=CARTESIAN_POINT ( 'NONE',  ( -28.63011601220122415, -359.5698779088871788, -26.28906389436296109 ) ) ;
#12637=LINE ( 'NONE', #44749, #9768 ) ;
#12639=ORIENTED_EDGE ( 'NONE', *, *, #1776, .T. ) ;
#12678=ORIENTED_EDGE ( 'NONE', *, *, #40804, .T. ) ;
#12692=DIRECTION ( 'NONE',  ( 0.000000000000000000, 0.000000000000000000, 1.000000000000000000 ) ) ;
#12729=VECTOR ( 'NONE', #36000, 1000.000000000000000 ) ;
#12731=VERTEX_POINT ( 'NONE', #29240 ) ;
#12738=ORIENTED_EDGE ( 'NONE', *, *, #11477, .F. ) ;
#12744=EDGE_CURVE ( 'NONE', #32355, #31022, #16675, .T. ) ;
#12746=CARTESIAN_POINT ( 'NONE',  ( -775.4999999999993179, -544.8427095258973623, -350.0000000000000000 ) ) ;
#12756=CIRCLE ( 'NONE', #44484, 9.999999999999982236 ) ;
#12779=VERTEX_POINT ( 'NONE', #603 ) ;
#12785=CYLINDRICAL_SURFACE ( 'NONE', #25539, 18.00000000000001421 ) ;
#12786=CARTESIAN_POINT ( 'NONE',  ( -26.63011601220122060, 26.27639943461401018, 900.0000000000001137 ) ) ;
#12787=EDGE_CURVE ( 'NONE', #28399, #11791, #43087, .T. ) ;
#12800=CARTESIAN_POINT ( 'NONE',  ( 775.4999999999993179, -513.1383975375929367, -367.9999999999999432 ) ) ;
#12803=LINE ( 'NONE', #34271, #964 ) ;
#12808=CARTESIAN_POINT ( 'NONE',  ( -786.4999999999993179, -513.1383975375929367, -369.9999999999999432 ) ) ;
#12811=FACE_OUTER_BOUND ( 'NONE', #10466, .T. ) ;
#12828=ORIENTED_EDGE ( 'NONE', *, *, #8660, .F. ) ;
#12835=ORIENTED_EDGE ( 'NONE', *, *, #40510, .T. ) ;
#12846=CIRCLE ( 'NONE', #18763, 12.00000000000001066 ) ;
#12847=EDGE_CURVE ( 'NONE', #37198, #9279, #32243, .T. ) ;
#12867=ADVANCED_FACE ( 'NONE', ( #18393 ), #28549, .F. ) ;
#12879=ORIENTED_EDGE ( 'NONE', *, *, #9669, .F. ) ;
#12913=EDGE_LOOP ( 'NONE', ( #33250, #23393 ) ) ;
#12918=DIRECTION ( 'NONE',  ( 1.000000000000000000, -0.000000000000000000, -0.000000000000000000 ) ) ;
#12992=DIRECTION ( 'NONE',  ( -1.000000000000000000, -0.000000000000000000, -0.000000000000000000 ) ) ;
#13015=DIRECTION ( 'NONE',  ( 0.000000000000000000, 0.3826834323650838421, 0.9238795325112891810 ) ) ;
#13019=AXIS2_PLACEMENT_3D ( 'NONE', #27685, #34623, #13602 ) ;
#13022=ORIENTED_EDGE ( 'NONE', *, *, #18304, .T. ) ;
#13054=CARTESIAN_POINT ( 'NONE',  ( -26.63011601220122060, -512.9681489794448908, -339.9999999999999432 ) ) ;
#13096=CARTESIAN_POINT ( 'NONE',  ( -26.63011601220122060, -513.1383975375929367, -369.9999999999999432 ) ) ;
#13133=DIRECTION ( 'NONE',  ( 1.000000000000000000, 0.000000000000000000, 0.000000000000000000 ) ) ;
#13152=AXIS2_PLACEMENT_3D ( 'NONE', #14253, #18632, #36179 ) ;
#13173=PLANE ( 'NONE',  #32865 ) ;
#13190=ORIENTED_EDGE ( 'NONE', *, *, #14278, .T. ) ;
#13196=PRODUCT_DEFINITION ( 'UNKNOWN', '', #37863, #27486 ) ;
#13218=ORIENTED_EDGE ( 'NONE', *, *, #36564, .F. ) ;
#13221=AXIS2_PLACEMENT_3D ( 'NONE', #11352, #32603, #29374 ) ;
#13243=ORIENTED_EDGE ( 'NONE', *, *, #4401, .T. ) ;
#13291=EDGE_CURVE ( 'NONE', #32281, #28399, #33153, .T. ) ;
#13335=EDGE_CURVE ( 'NONE', #36781, #2171, #11570, .T. ) ;
#13354=CARTESIAN_POINT ( 'NONE',  ( -746.4999999999993179, -365.3551492539851893, -18.13243251470705886 ) ) ;
#13362=ORIENTED_EDGE ( 'NONE', *, *, #15926, .T. ) ;
#13363=VERTEX_POINT ( 'NONE', #15588 ) ;
#13422=EDGE_LOOP ( 'NONE', ( #8784, #35897, #18691, #40870 ) ) ;
#13432=ORIENTED_EDGE ( 'NONE', *, *, #41613, .T. ) ;
#13435=CARTESIAN_POINT ( 'NONE',  ( -37.63011601220122770, -513.1383975375929367, -369.9999999999999432 ) ) ;
#13439=ORIENTED_EDGE ( 'NONE', *, *, #39900, .F. ) ;
#13446=EDGE_CURVE ( 'NONE', #15113, #29224, #4897, .T. ) ;
#13474=CARTESIAN_POINT ( 'NONE',  ( -786.4999999999993179, -32.84703287382745174, 757.2634078669104838 ) ) ;
#13502=EDGE_CURVE ( 'NONE', #36535, #30501, #3086, .T. ) ;
#13506=PLANE ( 'NONE',  #348 ) ;
#13509=DIRECTION ( 'NONE',  ( -1.000000000000000000, -0.000000000000000000, -0.000000000000000000 ) ) ;
#13545=LINE ( 'NONE', #2918, #40273 ) ;
#13553=MECHANICAL_DESIGN_GEOMETRIC_PRESENTATION_REPRESENTATION('',(#16474),#44500);
#13579=DIRECTION ( 'NONE',  ( 1.000000000000000000, -0.000000000000000000, -0.000000000000000000 ) ) ;
#13602=DIRECTION ( 'NONE',  ( 0.000000000000000000, 0.000000000000000000, 1.000000000000000000 ) ) ;
#13640=ADVANCED_FACE ( 'NONE', ( #34727 ), #38658, .T. ) ;
#13664=( GEOMETRIC_REPRESENTATION_CONTEXT ( 3 ) GLOBAL_UNCERTAINTY_ASSIGNED_CONTEXT ( ( #7979 ) ) GLOBAL_UNIT_ASSIGNED_CONTEXT ( ( #38802, #39253, #18005 ) ) REPRESENTATION_CONTEXT ( 'NONE', 'WORKASPACE' ) );
#13676=AXIS2_PLACEMENT_3D ( 'NONE', #31786, #30715, #32013 ) ;
#13704=CARTESIAN_POINT ( 'NONE',  ( -37.63011601220122770, -501.1515549466498669, -368.0974687824633520 ) ) ;
#13725=ORIENTED_EDGE ( 'NONE', *, *, #12847, .T. ) ;
#13737=DIRECTION ( 'NONE',  ( 0.000000000000000000, 0.000000000000000000, 1.000000000000000000 ) ) ;
#13740=DIRECTION ( 'NONE',  ( 0.000000000000000000, 0.3826834323650836756, 0.9238795325112892920 ) ) ;
#13755=VECTOR ( 'NONE', #25629, 1000.000000000000000 ) ;
#13789=AXIS2_PLACEMENT_3D ( 'NONE', #877, #11281, #21910 ) ;
#13792=AXIS2_PLACEMENT_3D ( 'NONE', #33533, #22682, #19221 ) ;
#13902=DIRECTION ( 'NONE',  ( 1.000000000000000000, 0.000000000000000000, 0.000000000000000000 ) ) ;
#13909=AXIS2_PLACEMENT_3D ( 'NONE', #7103, #34107, #6633 ) ;
#13914=ADVANCED_FACE ( 'NONE', ( #4005 ), #36723, .F. ) ;
#13923=DIRECTION ( 'NONE',  ( 0.000000000000000000, 0.000000000000000000, -1.000000000000000000 ) ) ;
#13925=ORIENTED_EDGE ( 'NONE', *, *, #17371, .F. ) ;
#13932=ORIENTED_EDGE ( 'NONE', *, *, #23265, .F. ) ;
#13934=ORIENTED_EDGE ( 'NONE', *, *, #29702, .F. ) ;
#13937=EDGE_LOOP ( 'NONE', ( #7058, #36807, #3376, #17272, #2863, #4914, #12835, #2912, #34704, #6768, #171, #9339 ) ) ;
#13940=ORIENTED_EDGE ( 'NONE', *, *, #2313, .T. ) ;
#13946=DIRECTION ( 'NONE',  ( 0.000000000000000000, 0.6755902076156502511, 0.7372773368101330771 ) ) ;
#13958=CARTESIAN_POINT ( 'NONE',  ( 786.4999999999993179, -32.84703287382739489, 757.2634078669103701 ) ) ;
#13959=FACE_BOUND ( 'NONE', #29557, .T. ) ;
#13979=VECTOR ( 'NONE', #30253, 1000.000000000000000 ) ;
#13980=CARTESIAN_POINT ( 'NONE',  ( -784.4999999999993179, -544.8427095258973623, -369.9999999999999432 ) ) ;
#14000=ORIENTED_EDGE ( 'NONE', *, *, #6611, .T. ) ;
#14031=CARTESIAN_POINT ( 'NONE',  ( -66.63011601220125613, -355.4967352946684969, -16.45562775363632113 ) ) ;
#14048=ORIENTED_EDGE ( 'NONE', *, *, #37141, .T. ) ;
#14054=ORIENTED_EDGE ( 'NONE', *, *, #2947, .T. ) ;
#14086=CARTESIAN_POINT ( 'NONE',  ( -28.63011601220122415, -512.9681489794448908, -339.9999999999999432 ) ) ;
#14114=CARTESIAN_POINT ( 'NONE',  ( -775.4999999999993179, -544.8427095258973623, -369.9999999999999432 ) ) ;
#14119=ORIENTED_EDGE ( 'NONE', *, *, #15376, .T. ) ;
#14122=DIRECTION ( 'NONE',  ( 0.000000000000000000, 0.3826834323650838421, 0.9238795325112891810 ) ) ;
#14146=LINE ( 'NONE', #11772, #7060 ) ;
#14228=ORIENTED_EDGE ( 'NONE', *, *, #20764, .F. ) ;
#14239=CARTESIAN_POINT ( 'NONE',  ( -773.4999999999993179, -513.1383975375929367, -369.9999999999999432 ) ) ;
#14246=LINE ( 'NONE', #44571, #39514 ) ;
#14253=CARTESIAN_POINT ( 'NONE',  ( 786.4999999999993179, -494.6608068873671300, -357.6536686473015720 ) ) ;
#14275=ORIENTED_EDGE ( 'NONE', *, *, #15051, .T. ) ;
#14278=EDGE_CURVE ( 'NONE', #1429, #16430, #20973, .T. ) ;
#14297=VERTEX_POINT ( 'NONE', #28613 ) ;
#14299=AXIS2_PLACEMENT_3D ( 'NONE', #24860, #43333, #38977 ) ;
#14301=AXIS2_PLACEMENT_3D ( 'NONE', #4854, #33050, #29355 ) ;
#14330=VECTOR ( 'NONE', #29914, 999.9999999999998863 ) ;
#14340=EDGE_LOOP ( 'NONE', ( #35232, #8951, #31012, #27389 ) ) ;
#14349=VERTEX_POINT ( 'NONE', #17069 ) ;
#14358=CIRCLE ( 'NONE', #35749, 12.00000000000001066 ) ;
#14362=AXIS2_PLACEMENT_3D ( 'NONE', #2587, #36793, #44169 ) ;
#14377=CIRCLE ( 'NONE', #40905, 9.999999999999980460 ) ;
#14383=VECTOR ( 'NONE', #4270, 1000.000000000000000 ) ;
#14405=CYLINDRICAL_SURFACE ( 'NONE', #22555, 9.999999999999980460 ) ;
#14407=ORIENTED_EDGE ( 'NONE', *, *, #44162, .T. ) ;
#14413=VECTOR ( 'NONE', #21404, 1000.000000000000114 ) ;
#14421=VECTOR ( 'NONE', #34534, 1000.000000000000000 ) ;
#14425=FACE_OUTER_BOUND ( 'NONE', #16829, .T. ) ;
#14479=VECTOR ( 'NONE', #13740, 1000.000000000000114 ) ;
#14480=PLANE ( 'NONE',  #34468 ) ;
#14496=PRODUCT_DEFINITION_SHAPE ( 'NONE', 'NONE',  #13196 ) ;
#14497=DIRECTION ( 'NONE',  ( -1.000000000000000000, -0.000000000000000000, -0.000000000000000000 ) ) ;
#14505=EDGE_CURVE ( 'NONE', #29708, #39647, #10832, .T. ) ;
#14513=AXIS2_PLACEMENT_3D ( 'NONE', #41900, #2635, #27565 ) ;
#14544=DIRECTION ( 'NONE',  ( 0.000000000000000000, 0.000000000000000000, 1.000000000000000000 ) ) ;
#14545=EDGE_CURVE ( 'NONE', #1111, #23251, #7593, .T. ) ;
#14562=EDGE_CURVE ( 'NONE', #34298, #30700, #21220, .T. ) ;
#14573=DIRECTION ( 'NONE',  ( -1.000000000000000000, -0.000000000000000000, -0.000000000000000000 ) ) ;
#14585=ORIENTED_EDGE ( 'NONE', *, *, #27442, .T. ) ;
#14603=DIRECTION ( 'NONE',  ( 0.000000000000000000, 0.3826834323650836200, 0.9238795325112892920 ) ) ;
#14608=CARTESIAN_POINT ( 'NONE',  ( -37.63011601220122770, -512.9681489794448908, -339.9999999999999432 ) ) ;
#14640=EDGE_LOOP ( 'NONE', ( #11264, #14585, #12639, #40415 ) ) ;
#14694=ORIENTED_EDGE ( 'NONE', *, *, #30089, .F. ) ;
#14704=CARTESIAN_POINT ( 'NONE',  ( -786.4999999999993179, -512.9681489794448908, -350.0000000000000000 ) ) ;
#14720=AXIS2_PLACEMENT_3D ( 'NONE', #14086, #31403, #7163 ) ;
#14726=CARTESIAN_POINT ( 'NONE',  ( 773.4999999999993179, -365.3551492539851893, -8.132432514707076621 ) ) ;
#14732=CARTESIAN_POINT ( 'NONE',  ( 1007.605605532488426, -112.8054336623104348, 752.6593748957919843 ) ) ;
#14739=ORIENTED_EDGE ( 'NONE', *, *, #10609, .T. ) ;
#14745=AXIS2_PLACEMENT_3D ( 'NONE', #12786, #39466, #18898 ) ;
#14758=CARTESIAN_POINT ( 'NONE',  ( 786.4999999999993179, -544.8427095258973623, -350.0000000000000000 ) ) ;
#14759=ORIENTED_EDGE ( 'NONE', *, *, #17608, .F. ) ;
#14769=ORIENTED_EDGE ( 'NONE', *, *, #8604, .T. ) ;
#14830=DIRECTION ( 'NONE',  ( 1.000000000000000000, -0.000000000000000000, -0.000000000000000000 ) ) ;
#14874=ORIENTED_EDGE ( 'NONE', *, *, #44060, .F. ) ;
#14884=LINE ( 'NONE', #43271, #24626 ) ;
#14895=DIRECTION ( 'NONE',  ( 0.000000000000000000, 0.9238795325112891810, -0.3826834323650838421 ) ) ;
#14899=EDGE_LOOP ( 'NONE', ( #13362, #17972, #1535, #10186 ) ) ;
#14917=FACE_OUTER_BOUND ( 'NONE', #20214, .T. ) ;
#14918=DIRECTION ( 'NONE',  ( 1.000000000000000000, 0.000000000000000000, 0.000000000000000000 ) ) ;
#14941=FACE_OUTER_BOUND ( 'NONE', #10873, .T. ) ;
#14943=AXIS2_PLACEMENT_3D ( 'NONE', #18177, #18401, #7543 ) ;
#14953=DIRECTION ( 'NONE',  ( 1.000000000000000000, 0.000000000000000000, -0.000000000000000000 ) ) ;
#14956=ORIENTED_EDGE ( 'NONE', *, *, #132, .F. ) ;
#14962=VERTEX_POINT ( 'NONE', #11283 ) ;
#15007=AXIS2_PLACEMENT_3D ( 'NONE', #38993, #13579, #27658 ) ;
#15032=EDGE_LOOP ( 'NONE', ( #16313, #2561, #5751, #31806, #29396, #41934, #38897, #19945 ) ) ;
#15041=( NAMED_UNIT ( * ) PLANE_ANGLE_UNIT ( ) SI_UNIT ( $, .RADIAN. ) );
#15051=EDGE_CURVE ( 'NONE', #25954, #463, #5248, .T. ) ;
#15063=EDGE_LOOP ( 'NONE', ( #29111, #14739, #12678, #37397 ) ) ;
#15088=AXIS2_PLACEMENT_3D ( 'NONE', #39128, #3085, #20854 ) ;
#15091=ORIENTED_EDGE ( 'NONE', *, *, #37961, .T. ) ;
#15113=VERTEX_POINT ( 'NONE', #12636 ) ;
#15125=STYLED_ITEM('',(#45758),#3320);
#15136=ORIENTED_EDGE ( 'NONE', *, *, #42455, .F. ) ;
#15146=CARTESIAN_POINT ( 'NONE',  ( -775.4999999999993179, -513.1383975375929367, -349.9999999999999432 ) ) ;
#15168=EDGE_CURVE ( 'NONE', #3612, #17065, #23014, .T. ) ;
#15173=FACE_OUTER_BOUND ( 'NONE', #36081, .T. ) ;
#15175=EDGE_CURVE ( 'NONE', #30803, #15113, #16105, .T. ) ;
#15215=CARTESIAN_POINT ( 'NONE',  ( -786.4999999999993179, -496.5085659523897448, -356.8883017825714319 ) ) ;
#15235=VECTOR ( 'NONE', #30810, 1000.000000000000000 ) ;
#15250=CIRCLE ( 'NONE', #13019, 18.00000000000001421 ) ;
#15262=VERTEX_POINT ( 'NONE', #37808 ) ;
#15264=LINE ( 'NONE', #15699, #6367 ) ;
#15266=AXIS2_PLACEMENT_3D ( 'NONE', #42877, #7786, #11478 ) ;
#15306=DIRECTION ( 'NONE',  ( 0.000000000000000000, 0.000000000000000000, 1.000000000000000000 ) ) ;
#15326=ORIENTED_EDGE ( 'NONE', *, *, #17347, .F. ) ;
#15329=DIRECTION ( 'NONE',  ( 1.000000000000000000, 0.000000000000000000, 0.000000000000000000 ) ) ;
#15339=AXIS2_PLACEMENT_3D ( 'NONE', #9550, #28006, #6998 ) ;
#15345=ORIENTED_EDGE ( 'NONE', *, *, #6009, .F. ) ;
#15374=DIRECTION ( 'NONE',  ( 1.000000000000000000, -0.000000000000000000, -0.000000000000000000 ) ) ;
#15375=CARTESIAN_POINT ( 'NONE',  ( -786.4999999999993179, -512.9681489794448908, -339.9999999999999432 ) ) ;
#15376=EDGE_CURVE ( 'NONE', #22437, #38191, #2463, .T. ) ;
#15407=EDGE_CURVE ( 'NONE', #41109, #26139, #21170, .T. ) ;
#15446=ADVANCED_FACE ( 'NONE', ( #23924 ), #14480, .F. ) ;
#15452=CARTESIAN_POINT ( 'NONE',  ( 1007.605605532488426, 26.27639943461424110, 900.0000000000004547 ) ) ;
#15525=ORIENTED_EDGE ( 'NONE', *, *, #12245, .T. ) ;
#15570=EDGE_CURVE ( 'NONE', #27963, #19960, #28088, .T. ) ;
#15571=ORIENTED_EDGE ( 'NONE', *, *, #31782, .F. ) ;
#15585=DIRECTION ( 'NONE',  ( 1.000000000000000000, -0.000000000000000000, -0.000000000000000000 ) ) ;
#15588=CARTESIAN_POINT ( 'NONE',  ( 784.4999999999993179, -512.9681489794448908, -352.0000000000000000 ) ) ;
#15596=DIRECTION ( 'NONE',  ( -0.000000000000000000, -0.3826834323650838421, -0.9238795325112891810 ) ) ;
#15612=DIRECTION ( 'NONE',  ( 0.000000000000000000, 0.000000000000000000, 1.000000000000000000 ) ) ;
#15651=LINE ( 'NONE', #29731, #20833 ) ;
#15665=EDGE_CURVE ( 'NONE', #44996, #24418, #38275, .T. ) ;
#15668=CARTESIAN_POINT ( 'NONE',  ( -775.4999999999993179, 22.32581219114657856, 895.6886905569881492 ) ) ;
#15681=EDGE_CURVE ( 'NONE', #17123, #38546, #23021, .T. ) ;
#15699=CARTESIAN_POINT ( 'NONE',  ( -26.63011601220122060, -496.5085659523897448, -356.8883017825714319 ) ) ;
#15720=CARTESIAN_POINT ( 'NONE',  ( -786.4999999999993179, 35.55895481007114967, 914.5706932916501728 ) ) ;
#15752=CIRCLE ( 'NONE', #27547, 12.00000000000001066 ) ;
#15802=CARTESIAN_POINT ( 'NONE',  ( -39.63011601220123481, -544.8427095258973623, -350.0000000000000000 ) ) ;
#15834=AXIS2_PLACEMENT_3D ( 'NONE', #22025, #7713, #318 ) ;
#15846=ORIENTED_EDGE ( 'NONE', *, *, #21942, .T. ) ;
#15864=VECTOR ( 'NONE', #2190, 1000.000000000000000 ) ;
#15880=ORIENTED_EDGE ( 'NONE', *, *, #11926, .T. ) ;
#15884=VECTOR ( 'NONE', #37076, 1000.000000000000114 ) ;
#15904=EDGE_CURVE ( 'NONE', #20268, #18154, #4309, .T. ) ;
#15910=ORIENTED_EDGE ( 'NONE', *, *, #35429, .T. ) ;
#15926=EDGE_CURVE ( 'NONE', #34816, #7814, #8010, .T. ) ;
#15930=EDGE_CURVE ( 'NONE', #1390, #43251, #909, .T. ) ;
#15933=ORIENTED_EDGE ( 'NONE', *, *, #36268, .F. ) ;
#15937=AXIS2_PLACEMENT_3D ( 'NONE', #15375, #15585, #29667 ) ;
#15941=CARTESIAN_POINT ( 'NONE',  ( -37.63011601220122770, -544.8427095258973623, -350.0000000000000000 ) ) ;
#16012=CARTESIAN_POINT ( 'NONE',  ( -786.4999999999993179, 22.32581219114657856, 895.6886905569881492 ) ) ;
#16034=EDGE_LOOP ( 'NONE', ( #37277, #37442, #34185, #15326 ) ) ;
#16050=LINE ( 'NONE', #24493, #36530 ) ;
#16069=FACE_OUTER_BOUND ( 'NONE', #30193, .T. ) ;
#16105=LINE ( 'NONE', #2008, #9386 ) ;
#16116=EDGE_LOOP ( 'NONE', ( #44247, #16135, #24932, #41671 ) ) ;
#16135=ORIENTED_EDGE ( 'NONE', *, *, #17396, .T. ) ;
#16139=EDGE_CURVE ( 'NONE', #42387, #37811, #9112, .T. ) ;
#16172=CARTESIAN_POINT ( 'NONE',  ( -775.4999999999993179, -544.8427095258973623, -369.9999999999999432 ) ) ;
#16180=DIRECTION ( 'NONE',  ( -1.000000000000000000, -0.000000000000000000, -0.000000000000000000 ) ) ;
#16221=PLANE ( 'NONE',  #43843 ) ;
#16252=ORIENTED_EDGE ( 'NONE', *, *, #30606, .F. ) ;
#16260=DIRECTION ( 'NONE',  ( 0.000000000000000000, 0.000000000000000000, 1.000000000000000000 ) ) ;
#16270=CARTESIAN_POINT ( 'NONE',  ( -784.4999999999993179, -501.1515549466498669, -368.0974687824633520 ) ) ;
#16276=DIRECTION ( 'NONE',  ( -1.000000000000000000, -0.000000000000000000, -0.000000000000000000 ) ) ;
#16279=LINE ( 'NONE', #15452, #552 ) ;
#16297=VERTEX_POINT ( 'NONE', #37751 ) ;
#16313=ORIENTED_EDGE ( 'NONE', *, *, #45051, .F. ) ;
#16318=DIRECTION ( 'NONE',  ( 0.000000000000000000, -0.9238795325112894030, 0.3826834323650836200 ) ) ;
#16326=CARTESIAN_POINT ( 'NONE',  ( 786.4999999999993179, -110.5936016518799221, 750.6326042729449455 ) ) ;
#16330=CARTESIAN_POINT ( 'NONE',  ( 784.4999999999993179, -359.5698779088871788, -26.28906389436296109 ) ) ;
#16341=CIRCLE ( 'NONE', #17106, 10.00000000000000888 ) ;
#16352=EDGE_CURVE ( 'NONE', #23251, #17287, #35553, .T. ) ;
#16430=VERTEX_POINT ( 'NONE', #24102 ) ;
#16454=CARTESIAN_POINT ( 'NONE',  ( -784.4999999999993179, -512.9681489794448908, -339.9999999999999432 ) ) ;
#16474=STYLED_ITEM('',(#45758),#33391);
#16480=ORIENTED_EDGE ( 'NONE', *, *, #27744, .T. ) ;
#16488=DIRECTION ( 'NONE',  ( 1.000000000000000000, -0.000000000000000000, -0.000000000000000000 ) ) ;
#16494=AXIS2_PLACEMENT_3D ( 'NONE', #5936, #30657, #44756 ) ;
#16495=VERTEX_POINT ( 'NONE', #13958 ) ;
#16505=CARTESIAN_POINT ( 'NONE',  ( -784.4999999999993179, -512.9681489794448908, -327.9999999999999432 ) ) ;
#16513=FACE_OUTER_BOUND ( 'NONE', #480, .T. ) ;
#16515=VECTOR ( 'NONE', #39353, 1000.000000000000114 ) ;
#16567=DIRECTION ( 'NONE',  ( -1.000000000000000000, -0.000000000000000000, -0.000000000000000000 ) ) ;
#16571=CIRCLE ( 'NONE', #15088, 19.99999999999990763 ) ;
#16579=EDGE_CURVE ( 'NONE', #38546, #30501, #33382, .T. ) ;
#16587=AXIS2_PLACEMENT_3D ( 'NONE', #42668, #39678, #7562 ) ;
#16633=DIRECTION ( 'NONE',  ( 0.000000000000000000, 0.000000000000000000, 1.000000000000000000 ) ) ;
#16639=CARTESIAN_POINT ( 'NONE',  ( -786.4999999999993179, -513.1383975375929367, -369.9999999999999432 ) ) ;
#16654=AXIS2_PLACEMENT_3D ( 'NONE', #18608, #43312, #10763 ) ;
#16675=CIRCLE ( 'NONE', #29951, 19.99999999999990763 ) ;
#16676=LINE ( 'NONE', #27292, #30758 ) ;
#16711=PLANE ( 'NONE',  #15339 ) ;
#16784=AXIS2_PLACEMENT_3D ( 'NONE', #8194, #7514, #7981 ) ;
#16813=ADVANCED_FACE ( 'NONE', ( #32650 ), #11853, .F. ) ;
#16818=VECTOR ( 'NONE', #34236, 1000.000000000000114 ) ;
#16829=EDGE_LOOP ( 'NONE', ( #14407, #23160, #15345, #1921 ) ) ;
#16830=ADVANCED_FACE ( 'NONE', ( #35884, #32193 ), #7954, .T. ) ;
#16856=ORIENTED_EDGE ( 'NONE', *, *, #38277, .T. ) ;
#16889=ORIENTED_EDGE ( 'NONE', *, *, #45565, .T. ) ;
#16922=CARTESIAN_POINT ( 'NONE',  ( -28.63011601220122415, -563.3203001761230553, -342.3463313526983143 ) ) ;
#16952=CARTESIAN_POINT ( 'NONE',  ( -786.4999999999993179, -563.3203001761230553, -342.3463313526983143 ) ) ;
#16954=VERTEX_POINT ( 'NONE', #993 ) ;
#16956=DIRECTION ( 'NONE',  ( -1.000000000000000000, -0.000000000000000000, -0.000000000000000000 ) ) ;
#16957=DIRECTION ( 'NONE',  ( -1.000000000000000000, -0.000000000000000000, -0.000000000000000000 ) ) ;
#17007=DIRECTION ( 'NONE',  ( -1.000000000000000000, -0.000000000000000000, -0.000000000000000000 ) ) ;
#17024=FACE_OUTER_BOUND ( 'NONE', #6699, .T. ) ;
#17040=ORIENTED_EDGE ( 'NONE', *, *, #23904, .F. ) ;
#17051=ORIENTED_EDGE ( 'NONE', *, *, #30056, .T. ) ;
#17065=VERTEX_POINT ( 'NONE', #33542 ) ;
#17069=CARTESIAN_POINT ( 'NONE',  ( 773.4999999999993179, -365.3551492539851893, -28.13243251470704109 ) ) ;
#17106=AXIS2_PLACEMENT_3D ( 'NONE', #24497, #13902, #3511 ) ;
#17108=VERTEX_POINT ( 'NONE', #36999 ) ;
#17120=DIRECTION ( 'NONE',  ( -0.000000000000000000, 0.6755902076156502511, 0.7372773368101330771 ) ) ;
#17123=VERTEX_POINT ( 'NONE', #40699 ) ;
#17134=AXIS2_PLACEMENT_3D ( 'NONE', #19280, #29906, #43991 ) ;
#17139=CARTESIAN_POINT ( 'NONE',  ( 786.4999999999993179, -512.9681489794448908, -339.9999999999999432 ) ) ;
#17152=VERTEX_POINT ( 'NONE', #23364 ) ;
#17166=AXIS2_PLACEMENT_3D ( 'NONE', #7710, #315, #32879 ) ;
#17172=CARTESIAN_POINT ( 'NONE',  ( 773.4999999999993179, -494.6608068873671300, -357.6536686473015720 ) ) ;
#17176=DIRECTION ( 'NONE',  ( 1.000000000000000000, -0.000000000000000000, -0.000000000000000000 ) ) ;
#17187=VECTOR ( 'NONE', #33831, 1000.000000000000114 ) ;
#17203=CARTESIAN_POINT ( 'NONE',  ( 786.4999999999993179, -365.3551492539851893, -28.13243251470704109 ) ) ;
#17210=CYLINDRICAL_SURFACE ( 'NONE', #1991, 9.999999999999980460 ) ;
#17237=CARTESIAN_POINT ( 'NONE',  ( -773.4999999999993179, -365.3551492539851893, -18.13243251470705886 ) ) ;
#17251=CARTESIAN_POINT ( 'NONE',  ( -786.4999999999993179, 26.27639943461424110, 900.0000000000004547 ) ) ;
#17252=PLANE ( 'NONE',  #13909 ) ;
#17254=AXIS2_PLACEMENT_3D ( 'NONE', #2651, #34969, #24339 ) ;
#17268=AXIS2_PLACEMENT_3D ( 'NONE', #29850, #40032, #36785 ) ;
#17272=ORIENTED_EDGE ( 'NONE', *, *, #7810, .F. ) ;
#17274=ORIENTED_EDGE ( 'NONE', *, *, #45466, .T. ) ;
#17285=AXIS2_PLACEMENT_3D ( 'NONE', #27518, #34688, #3517 ) ;
#17287=VERTEX_POINT ( 'NONE', #27976 ) ;
#17301=VECTOR ( 'NONE', #8098, 1000.000000000000000 ) ;
#17304=AXIS2_PLACEMENT_3D ( 'NONE', #7102, #17949, #22973 ) ;
#17326=UNCERTAINTY_MEASURE_WITH_UNIT (LENGTH_MEASURE( 1.000000000000000082E-05 ), #40357, 'distance_accuracy_value', 'NONE');
#17334=VECTOR ( 'NONE', #3169, 1000.000000000000000 ) ;
#17347=EDGE_CURVE ( 'NONE', #2958, #33261, #44860, .T. ) ;
#17371=EDGE_CURVE ( 'NONE', #34451, #1374, #16341, .T. ) ;
#17377=CARTESIAN_POINT ( 'NONE',  ( -775.4999999999993179, -513.1383975375929367, -367.9999999999999432 ) ) ;
#17393=ORIENTED_EDGE ( 'NONE', *, *, #35409, .T. ) ;
#17396=EDGE_CURVE ( 'NONE', #2677, #22833, #38382, .T. ) ;
#17399=AXIS2_PLACEMENT_3D ( 'NONE', #15146, #14918, #36374 ) ;
#17414=DIRECTION ( 'NONE',  ( 0.000000000000000000, 0.000000000000000000, 1.000000000000000000 ) ) ;
#17432=CARTESIAN_POINT ( 'NONE',  ( -775.4999999999993179, -512.9681489794448908, -352.0000000000000000 ) ) ;
#17480=VECTOR ( 'NONE', #11748, 1000.000000000000000 ) ;
#17489=CARTESIAN_POINT ( 'NONE',  ( -786.4999999999993179, -513.1383975375929367, -369.9999999999999432 ) ) ;
#17608=EDGE_CURVE ( 'NONE', #10339, #25758, #36279, .T. ) ;
#17646=EDGE_CURVE ( 'NONE', #34942, #31246, #260, .T. ) ;
#17688=DIRECTION ( 'NONE',  ( 0.000000000000000000, -0.3826834323650838421, -0.9238795325112891810 ) ) ;
#17697=MANIFOLD_SOLID_BREP ( 'Body-Move/Copy1', #30602 ) ;
#17716=CARTESIAN_POINT ( 'NONE',  ( 786.4999999999993179, -513.1383975375929367, -369.9999999999999432 ) ) ;
#17760=DIRECTION ( 'NONE',  ( -0.000000000000000000, 1.000000000000000000, -0.000000000000000000 ) ) ;
#17765=CARTESIAN_POINT ( 'NONE',  ( -37.63011601220122770, -501.1515549466498669, -368.0974687824633520 ) ) ;
#17782=DIRECTION ( 'NONE',  ( 1.000000000000000000, -0.000000000000000000, -0.000000000000000000 ) ) ;
#17806=ORIENTED_EDGE ( 'NONE', *, *, #4320, .T. ) ;
#17825=CARTESIAN_POINT ( 'NONE',  ( -37.63011601220122770, -365.3551492539851893, -18.13243251470705886 ) ) ;
#17864=CARTESIAN_POINT ( 'NONE',  ( -786.4999999999993179, -513.1383975375929367, -369.9999999999999432 ) ) ;
#17878=DIRECTION ( 'NONE',  ( -1.000000000000000000, -0.000000000000000000, 0.000000000000000000 ) ) ;
#17884=DIRECTION ( 'NONE',  ( 0.000000000000000000, 0.3826834323650836756, 0.9238795325112892920 ) ) ;
#17918=EDGE_CURVE ( 'NONE', #10012, #35031, #2291, .T. ) ;
#17949=DIRECTION ( 'NONE',  ( -1.000000000000000000, -0.000000000000000000, -0.000000000000000000 ) ) ;
#17950=DIRECTION ( 'NONE',  ( -1.000000000000000000, -0.000000000000000000, -0.000000000000000000 ) ) ;
#17970=ORIENTED_EDGE ( 'NONE', *, *, #29198, .F. ) ;
#17972=ORIENTED_EDGE ( 'NONE', *, *, #45351, .T. ) ;
#18005=( NAMED_UNIT ( * ) SI_UNIT ( $, .STERADIAN. ) SOLID_ANGLE_UNIT ( ) );
#18037=CARTESIAN_POINT ( 'NONE',  ( -26.63011601220122060, -563.3203001761230553, -342.3463313526983143 ) ) ;
#18054=DIRECTION ( 'NONE',  ( 0.000000000000000000, 0.000000000000000000, 1.000000000000000000 ) ) ;
#18057=CARTESIAN_POINT ( 'NONE',  ( 784.4999999999993179, -110.5936016518799221, 750.6326042729449455 ) ) ;
#18095=ORIENTED_EDGE ( 'NONE', *, *, #9669, .T. ) ;
#18100=FACE_OUTER_BOUND ( 'NONE', #27791, .T. ) ;
#18105=DIRECTION ( 'NONE',  ( 0.000000000000000000, 0.000000000000000000, 1.000000000000000000 ) ) ;
#18110=VECTOR ( 'NONE', #40102, 1000.000000000000000 ) ;
#18117=CARTESIAN_POINT ( 'NONE',  ( -786.4999999999993179, -512.9681489794448908, -352.0000000000000000 ) ) ;
#18144=ORIENTED_EDGE ( 'NONE', *, *, #32011, .F. ) ;
#18150=ADVANCED_FACE ( 'NONE', ( #19401, #36952 ), #26772, .F. ) ;
#18151=VECTOR ( 'NONE', #6828, 1000.000000000000114 ) ;
#18154=VERTEX_POINT ( 'NONE', #1833 ) ;
#18167=DIRECTION ( 'NONE',  ( 1.000000000000000000, 0.000000000000000000, 0.000000000000000000 ) ) ;
#18177=CARTESIAN_POINT ( 'NONE',  ( -784.4999999999993179, -512.9681489794448908, -339.9999999999999432 ) ) ;
#18210=AXIS2_PLACEMENT_3D ( 'NONE', #26711, #30648, #40383 ) ;
#18227=FACE_BOUND ( 'NONE', #8107, .T. ) ;
#18234=LINE ( 'NONE', #39241, #29744 ) ;
#18246=VECTOR ( 'NONE', #27921, 1000.000000000000000 ) ;
#18259=EDGE_CURVE ( 'NONE', #22319, #16495, #20077, .T. ) ;
#18271=DIRECTION ( 'NONE',  ( -1.000000000000000000, -0.000000000000000000, -0.000000000000000000 ) ) ;
#18294=DIRECTION ( 'NONE',  ( 0.000000000000000000, 0.000000000000000000, 1.000000000000000000 ) ) ;
#18304=EDGE_CURVE ( 'NONE', #33295, #24190, #33578, .T. ) ;
#18344=ORIENTED_EDGE ( 'NONE', *, *, #5817, .F. ) ;
#18350=CARTESIAN_POINT ( 'NONE',  ( 784.4999999999993179, -544.8427095258973623, -350.0000000000000000 ) ) ;
#18364=EDGE_CURVE ( 'NONE', #11223, #17152, #14246, .T. ) ;
#18367=DIRECTION ( 'NONE',  ( 0.000000000000000000, 0.000000000000000000, 1.000000000000000000 ) ) ;
#18393=FACE_OUTER_BOUND ( 'NONE', #24886, .T. ) ;
#18401=DIRECTION ( 'NONE',  ( 1.000000000000000000, 0.000000000000000000, 0.000000000000000000 ) ) ;
#18412=CARTESIAN_POINT ( 'NONE',  ( -773.4999999999993179, -494.6608068873671300, -357.6536686473015720 ) ) ;
#18420=EDGE_LOOP ( 'NONE', ( #33705, #25735, #44082, #3186, #16889, #10137 ) ) ;
#18434=AXIS2_PLACEMENT_3D ( 'NONE', #35989, #871, #7826 ) ;
#18458=ORIENTED_EDGE ( 'NONE', *, *, #39900, .T. ) ;
#18503=CARTESIAN_POINT ( 'NONE',  ( -37.63011601220122770, -512.9681489794448908, -339.9999999999999432 ) ) ;
#18516=ADVANCED_FACE ( 'NONE', ( #25304 ), #7768, .T. ) ;
#18557=DIRECTION ( 'NONE',  ( 0.000000000000000000, 0.000000000000000000, -1.000000000000000000 ) ) ;
#18589=ORIENTED_EDGE ( 'NONE', *, *, #36318, .T. ) ;
#18593=DIRECTION ( 'NONE',  ( 0.000000000000000000, 0.000000000000000000, 1.000000000000000000 ) ) ;
#18608=CARTESIAN_POINT ( 'NONE',  ( 786.4999999999993179, -513.1383975375929367, -369.9999999999999432 ) ) ;
#18612=DIRECTION ( 'NONE',  ( 0.000000000000000000, 0.000000000000000000, 1.000000000000000000 ) ) ;
#18631=DIRECTION ( 'NONE',  ( 0.000000000000000000, -0.6755902076156505842, -0.7372773368101328550 ) ) ;
#18632=DIRECTION ( 'NONE',  ( 0.000000000000000000, -0.9238795325112892920, 0.3826834323650836756 ) ) ;
#18662=FACE_OUTER_BOUND ( 'NONE', #15032, .T. ) ;
#18666=ORIENTED_EDGE ( 'NONE', *, *, #39030, .F. ) ;
#18684=CARTESIAN_POINT ( 'NONE',  ( -39.63011601220123481, -110.5936016518799221, 750.6326042729449455 ) ) ;
#18691=ORIENTED_EDGE ( 'NONE', *, *, #13335, .T. ) ;
#18702=EDGE_LOOP ( 'NONE', ( #33191, #42397, #27669, #25001, #24832, #43356 ) ) ;
#18721=CARTESIAN_POINT ( 'NONE',  ( 1007.605605532488426, -32.84703287382739489, 757.2634078669104838 ) ) ;
#18746=STYLED_ITEM('',(#45758),#1418);
#18763=AXIS2_PLACEMENT_3D ( 'NONE', #21932, #32082, #11540 ) ;
#18770=EDGE_LOOP ( 'NONE', ( #18458, #44718, #37144, #20040 ) ) ;
#18774=ORIENTED_EDGE ( 'NONE', *, *, #12744, .T. ) ;
#18821=DIRECTION ( 'NONE',  ( -1.000000000000000000, -0.000000000000000000, 0.000000000000000000 ) ) ;
#18823=ORIENTED_EDGE ( 'NONE', *, *, #38798, .T. ) ;
#18832=ORIENTED_EDGE ( 'NONE', *, *, #24955, .T. ) ;
#18837=DIRECTION ( 'NONE',  ( 0.000000000000000000, 0.000000000000000000, 1.000000000000000000 ) ) ;
#18842=ORIENTED_EDGE ( 'NONE', *, *, #19601, .F. ) ;
#18850=DIRECTION ( 'NONE',  ( 0.000000000000000000, -0.3826834323650836756, -0.9238795325112892920 ) ) ;
#18857=FACE_OUTER_BOUND ( 'NONE', #10569, .T. ) ;
#18873=ORIENTED_EDGE ( 'NONE', *, *, #27521, .F. ) ;
#18885=ORIENTED_EDGE ( 'NONE', *, *, #35330, .T. ) ;
#18898=DIRECTION ( 'NONE',  ( 0.000000000000000000, 0.6755902076156505842, 0.7372773368101327440 ) ) ;
#18900=CYLINDRICAL_SURFACE ( 'NONE', #36546, 18.00000000000001421 ) ;
#18905=LINE ( 'NONE', #8270, #26293 ) ;
#18909=AXIS2_PLACEMENT_3D ( 'NONE', #15802, #37041, #18837 ) ;
#18927=ORIENTED_EDGE ( 'NONE', *, *, #10609, .F. ) ;
#18932=LINE ( 'NONE', #3533, #13755 ) ;
#18972=DIRECTION ( 'NONE',  ( 0.000000000000000000, 0.000000000000000000, 1.000000000000000000 ) ) ;
#18985=AXIS2_PLACEMENT_3D ( 'NONE', #9117, #29316, #34275 ) ;
#18996=ORIENTED_EDGE ( 'NONE', *, *, #10845, .F. ) ;
#19003=VERTEX_POINT ( 'NONE', #12800 ) ;
#19014=CARTESIAN_POINT ( 'NONE',  ( -786.4999999999993179, -494.6608068873671300, -357.6536686473015720 ) ) ;
#19020=CARTESIAN_POINT ( 'NONE',  ( -26.63011601220122060, 26.27639943461401018, 900.0000000000001137 ) ) ;
#19038=ORIENTED_EDGE ( 'NONE', *, *, #45342, .F. ) ;
#19043=ADVANCED_FACE ( 'NONE', ( #33597, #10193 ), #45546, .T. ) ;
#19044=EDGE_LOOP ( 'NONE', ( #37679, #20127 ) ) ;
#19069=ADVANCED_FACE ( 'NONE', ( #31662 ), #42067, .F. ) ;
#19077=EDGE_CURVE ( 'NONE', #5018, #7856, #16050, .T. ) ;
#19079=PLANE ( 'NONE',  #33465 ) ;
#19116=DIRECTION ( 'NONE',  ( 0.000000000000000000, 0.6755902076156505842, 0.7372773368101327440 ) ) ;
#19148=FACE_OUTER_BOUND ( 'NONE', #29946, .T. ) ;
#19157=ORIENTED_EDGE ( 'NONE', *, *, #32264, .T. ) ;
#19204=CARTESIAN_POINT ( 'NONE',  ( 784.4999999999993179, -513.1383975375929367, -349.9999999999999432 ) ) ;
#19208=ORIENTED_EDGE ( 'NONE', *, *, #36564, .T. ) ;
#19221=DIRECTION ( 'NONE',  ( 0.000000000000000000, 0.000000000000000000, -1.000000000000000000 ) ) ;
#19224=ORIENTED_EDGE ( 'NONE', *, *, #43262, .F. ) ;
#19232=CARTESIAN_POINT ( 'NONE',  ( 746.4999999999993179, -365.3551492539851893, -28.13243251470704109 ) ) ;
#19266=CARTESIAN_POINT ( 'NONE',  ( -66.63011601220125613, -365.3551492539851893, -28.13243251470704109 ) ) ;
#19268=ADVANCED_FACE ( 'NONE', ( #9110 ), #24270, .F. ) ;
#19280=CARTESIAN_POINT ( 'NONE',  ( 773.4999999999993179, -512.9681489794448908, -339.9999999999999432 ) ) ;
#19295=PLANE ( 'NONE',  #37946 ) ;
#19300=DIRECTION ( 'NONE',  ( 1.000000000000000000, 0.000000000000000000, -0.000000000000000000 ) ) ;
#19308=STYLED_ITEM('',(#45758),#17697);
#19312=ORIENTED_EDGE ( 'NONE', *, *, #38068, .F. ) ;
#19320=EDGE_LOOP ( 'NONE', ( #1206, #11379, #10232, #44196 ) ) ;
#19325=EDGE_CURVE ( 'NONE', #15262, #2064, #40606, .T. ) ;
#19338=DIRECTION ( 'NONE',  ( 0.000000000000000000, 0.3826834323650836756, 0.9238795325112892920 ) ) ;
#19341=VERTEX_POINT ( 'NONE', #21735 ) ;
#19392=ORIENTED_EDGE ( 'NONE', *, *, #20155, .F. ) ;
#19394=AXIS2_PLACEMENT_3D ( 'NONE', #21399, #32007, #28309 ) ;
#19401=FACE_OUTER_BOUND ( 'NONE', #41530, .T. ) ;
#19422=AXIS2_PLACEMENT_3D ( 'NONE', #40391, #1559, #20026 ) ;
#19423=DIRECTION ( 'NONE',  ( 0.000000000000000000, 0.7372773368101331881, -0.6755902076156503622 ) ) ;
#19477=EDGE_LOOP ( 'NONE', ( #37500, #13218, #32764, #35395 ) ) ;
#19489=DIRECTION ( 'NONE',  ( -1.000000000000000000, -0.000000000000000000, -0.000000000000000000 ) ) ;
#19490=ORIENTED_EDGE ( 'NONE', *, *, #22946, .F. ) ;
#19496=VECTOR ( 'NONE', #18271, 1000.000000000000000 ) ;
#19508=LINE ( 'NONE', #1718, #14330 ) ;
#19538=VECTOR ( 'NONE', #40283, 1000.000000000000000 ) ;
#19543=VERTEX_POINT ( 'NONE', #17251 ) ;
#19558=CARTESIAN_POINT ( 'NONE',  ( 786.4999999999993179, -513.1383975375929367, -369.9999999999999432 ) ) ;
#19559=PLANE ( 'NONE',  #1243 ) ;
#19573=VECTOR ( 'NONE', #11655, 999.9999999999998863 ) ;
#19577=VERTEX_POINT ( 'NONE', #38055 ) ;
#19584=ORIENTED_EDGE ( 'NONE', *, *, #14562, .T. ) ;
#19587=CARTESIAN_POINT ( 'NONE',  ( -37.63011601220122770, -513.1383975375929367, -367.9999999999999432 ) ) ;
#19597=ORIENTED_EDGE ( 'NONE', *, *, #23222, .F. ) ;
#19600=VECTOR ( 'NONE', #36350, 1000.000000000000114 ) ;
#19601=EDGE_CURVE ( 'NONE', #38191, #3542, #37749, .T. ) ;
#19636=VECTOR ( 'NONE', #37599, 999.9999999999998863 ) ;
#19737=VECTOR ( 'NONE', #23097, 1000.000000000000114 ) ;
#19741=DIRECTION ( 'NONE',  ( 1.000000000000000000, 0.000000000000000000, 0.000000000000000000 ) ) ;
#19751=CARTESIAN_POINT ( 'NONE',  ( -37.63011601220122770, -857.0166862835568509, -63.94525337997358605 ) ) ;
#19795=DIRECTION ( 'NONE',  ( 0.000000000000000000, -0.3826834323650838976, -0.9238795325112892920 ) ) ;
#19821=CARTESIAN_POINT ( 'NONE',  ( -773.4999999999993179, -110.5936016518799221, 750.6326042729449455 ) ) ;
#19832=CIRCLE ( 'NONE', #31609, 10.00000000000000888 ) ;
#19836=EDGE_CURVE ( 'NONE', #5018, #2958, #37007, .T. ) ;
#19850=ADVANCED_FACE ( 'NONE', ( #27641 ), #35262, .F. ) ;
#19906=CARTESIAN_POINT ( 'NONE',  ( -26.63011601220122060, -110.5936016518799221, 750.6326042729449455 ) ) ;
#19909=ORIENTED_EDGE ( 'NONE', *, *, #28592, .T. ) ;
#19916=LINE ( 'NONE', #27079, #4161 ) ;
#19921=EDGE_CURVE ( 'NONE', #7984, #30278, #35714, .T. ) ;
#19945=ORIENTED_EDGE ( 'NONE', *, *, #35429, .F. ) ;
#19957=DIRECTION ( 'NONE',  ( -1.000000000000000000, -0.000000000000000000, -0.000000000000000000 ) ) ;
#19960=VERTEX_POINT ( 'NONE', #21865 ) ;
#19962=CARTESIAN_POINT ( 'NONE',  ( 786.4999999999993179, -512.9681489794448908, -352.0000000000000000 ) ) ;
#20017=CARTESIAN_POINT ( 'NONE',  ( 784.4999999999993179, -544.8427095258973623, -369.9999999999999432 ) ) ;
#20026=DIRECTION ( 'NONE',  ( 0.000000000000000000, 0.000000000000000000, 1.000000000000000000 ) ) ;
#20040=ORIENTED_EDGE ( 'NONE', *, *, #42114, .T. ) ;
#20069=EDGE_CURVE ( 'NONE', #39647, #2064, #161, .T. ) ;
#20077=LINE ( 'NONE', #35478, #14413 ) ;
#20096=DIRECTION ( 'NONE',  ( 0.000000000000000000, 0.000000000000000000, 1.000000000000000000 ) ) ;
#20118=CIRCLE ( 'NONE', #19394, 9.999999999999982236 ) ;
#20120=ORIENTED_EDGE ( 'NONE', *, *, #28077, .T. ) ;
#20127=ORIENTED_EDGE ( 'NONE', *, *, #38295, .T. ) ;
#20136=PLANE ( 'NONE',  #14362 ) ;
#20142=EDGE_CURVE ( 'NONE', #39064, #21254, #45679, .T. ) ;
#20143=DIRECTION ( 'NONE',  ( 0.000000000000000000, -0.3826834323650838976, -0.9238795325112892920 ) ) ;
#20155=EDGE_CURVE ( 'NONE', #20268, #4067, #20989, .T. ) ;
#20170=ADVANCED_FACE ( 'NONE', ( #15173 ), #19295, .F. ) ;
#20176=LINE ( 'NONE', #16952, #15235 ) ;
#20177=LINE ( 'NONE', #23853, #10307 ) ;
#20186=DIRECTION ( 'NONE',  ( 0.000000000000000000, -0.3826834323650835645, -0.9238795325112892920 ) ) ;
#20205=CARTESIAN_POINT ( 'NONE',  ( -786.4999999999993179, -544.8427095258973623, -369.9999999999999432 ) ) ;
#20214=EDGE_LOOP ( 'NONE', ( #15525, #21332, #22426, #1743 ) ) ;
#20263=AXIS2_PLACEMENT_3D ( 'NONE', #42205, #31116, #31585 ) ;
#20266=DIRECTION ( 'NONE',  ( 0.000000000000000000, -0.6755902076156505842, -0.7372773368101327440 ) ) ;
#20268=VERTEX_POINT ( 'NONE', #26675 ) ;
#20297=VECTOR ( 'NONE', #44937, 1000.000000000000000 ) ;
#20311=CIRCLE ( 'NONE', #30645, 9.999999999999982236 ) ;
#20404=DIRECTION ( 'NONE',  ( 1.000000000000000000, -0.000000000000000000, -0.000000000000000000 ) ) ;
#20427=DIRECTION ( 'NONE',  ( 0.000000000000000000, 0.7372773368101421809, -0.6755902076156404812 ) ) ;
#20431=CARTESIAN_POINT ( 'NONE',  ( -37.63011601220122770, -544.8427095258973623, -369.9999999999999432 ) ) ;
#20446=EDGE_CURVE ( 'NONE', #24418, #17108, #8457, .T. ) ;
#20475=EDGE_CURVE ( 'NONE', #37268, #28399, #22301, .T. ) ;
#20495=DIRECTION ( 'NONE',  ( 0.000000000000000000, 0.000000000000000000, -1.000000000000000000 ) ) ;
#20595=CARTESIAN_POINT ( 'NONE',  ( -786.4999999999993179, -512.9681489794448908, -350.0000000000000000 ) ) ;
#20641=CYLINDRICAL_SURFACE ( 'NONE', #5398, 20.00000000000001776 ) ;
#20648=CARTESIAN_POINT ( 'NONE',  ( -775.4999999999993179, -501.1515549466498669, -368.0974687824633520 ) ) ;
#20655=LINE ( 'NONE', #20205, #6951 ) ;
#20764=EDGE_CURVE ( 'NONE', #5117, #44956, #40908, .T. ) ;
#20771=EDGE_CURVE ( 'NONE', #34249, #31022, #20655, .T. ) ;
#20833=VECTOR ( 'NONE', #33002, 1000.000000000000114 ) ;
#20854=DIRECTION ( 'NONE',  ( 0.000000000000000000, 0.000000000000000000, 1.000000000000000000 ) ) ;
#20891=PLANE ( 'NONE',  #25343 ) ;
#20911=ORIENTED_EDGE ( 'NONE', *, *, #23265, .T. ) ;
#20960=AXIS2_PLACEMENT_3D ( 'NONE', #7259, #6778, #31713 ) ;
#20973=LINE ( 'NONE', #6670, #45529 ) ;
#20989=CIRCLE ( 'NONE', #17304, 9.999999999999982236 ) ;
#21002=MECHANICAL_DESIGN_GEOMETRIC_PRESENTATION_REPRESENTATION('',(#15125),#13664);
#21038=EDGE_LOOP ( 'NONE', ( #43422, #28235, #41823, #11375 ) ) ;
#21041=CARTESIAN_POINT ( 'NONE',  ( -26.63011601220122060, -513.1383975375929367, -369.9999999999999432 ) ) ;
#21046=DIRECTION ( 'NONE',  ( -1.000000000000000000, -0.000000000000000000, -0.000000000000000000 ) ) ;
#21080=CIRCLE ( 'NONE', #44691, 20.00000000000001776 ) ;
#21098=EDGE_CURVE ( 'NONE', #34451, #29646, #39148, .T. ) ;
#21113=DIRECTION ( 'NONE',  ( 0.000000000000000000, 0.000000000000000000, 1.000000000000000000 ) ) ;
#21155=FACE_BOUND ( 'NONE', #43730, .T. ) ;
#21170=LINE ( 'NONE', #17716, #28583 ) ;
#21220=LINE ( 'NONE', #17765, #7924 ) ;
#21254=VERTEX_POINT ( 'NONE', #21802 ) ;
#21258=EDGE_CURVE ( 'NONE', #10285, #19003, #3800, .T. ) ;
#21278=EDGE_CURVE ( 'NONE', #13363, #40120, #7757, .T. ) ;
#21287=AXIS2_PLACEMENT_3D ( 'NONE', #41622, #24283, #6738 ) ;
#21289=LINE ( 'NONE', #41861, #23481 ) ;
#21315=EDGE_CURVE ( 'NONE', #7478, #33715, #1240, .T. ) ;
#21326=DIRECTION ( 'NONE',  ( 1.000000000000000000, 0.000000000000000000, -0.000000000000000000 ) ) ;
#21332=ORIENTED_EDGE ( 'NONE', *, *, #11685, .T. ) ;
#21335=CARTESIAN_POINT ( 'NONE',  ( -786.4999999999993179, -292.9981031064102126, 121.3637880562633171 ) ) ;
#21358=EDGE_CURVE ( 'NONE', #31246, #19577, #33326, .T. ) ;
#21399=CARTESIAN_POINT ( 'NONE',  ( -39.63011601220123481, -365.3551492539851893, -18.13243251470705886 ) ) ;
#21404=DIRECTION ( 'NONE',  ( 0.000000000000000000, -0.3826834323650837866, -0.9238795325112891810 ) ) ;
#21491=DIRECTION ( 'NONE',  ( 0.000000000000000000, 0.000000000000000000, 1.000000000000000000 ) ) ;
#21516=VECTOR ( 'NONE', #6730, 1000.000000000000000 ) ;
#21561=LINE ( 'NONE', #11401, #43151 ) ;
#21577=CARTESIAN_POINT ( 'NONE',  ( 786.4999999999993179, 323.4107432173689176, 352.9408934102648345 ) ) ;
#21598=ORIENTED_EDGE ( 'NONE', *, *, #43293, .T. ) ;
#21622=ADVANCED_FACE ( 'NONE', ( #36020, #16069, #1517 ), #30609, .T. ) ;
#21675=AXIS2_PLACEMENT_3D ( 'NONE', #24174, #3157, #10320 ) ;
#21685=VECTOR ( 'NONE', #7708, 1000.000000000000114 ) ;
#21719=LINE ( 'NONE', #35813, #3941 ) ;
#21729=CARTESIAN_POINT ( 'NONE',  ( -786.4999999999993179, -365.3551492539851893, -18.13243251470705886 ) ) ;
#21735=CARTESIAN_POINT ( 'NONE',  ( -784.4999999999993179, -496.5085659523897448, -356.8883017825714319 ) ) ;
#21737=CARTESIAN_POINT ( 'NONE',  ( -39.63011601220123481, -365.3551492539851893, -8.132432514707076621 ) ) ;
#21751=VECTOR ( 'NONE', #4544, 1000.000000000000000 ) ;
#21783=DIRECTION ( 'NONE',  ( 1.000000000000000000, 0.000000000000000000, -0.000000000000000000 ) ) ;
#21802=CARTESIAN_POINT ( 'NONE',  ( 775.4999999999993179, -496.5085659523897448, -356.8883017825714319 ) ) ;
#21817=DIRECTION ( 'NONE',  ( 0.000000000000000000, 0.000000000000000000, -1.000000000000000000 ) ) ;
#21833=CARTESIAN_POINT ( 'NONE',  ( 775.4999999999993179, -563.3203001761231690, -342.3463313526983143 ) ) ;
#21836=EDGE_CURVE ( 'NONE', #29708, #15262, #5670, .T. ) ;
#21843=DIRECTION ( 'NONE',  ( 0.000000000000000000, 0.000000000000000000, 1.000000000000000000 ) ) ;
#21849=CARTESIAN_POINT ( 'NONE',  ( -775.4999999999993179, -563.3203001761231690, -342.3463313526983143 ) ) ;
#21864=CIRCLE ( 'NONE', #1926, 10.00000000000000888 ) ;
#21865=CARTESIAN_POINT ( 'NONE',  ( -773.4999999999993179, -513.1383975375929367, -369.9999999999999432 ) ) ;
#21872=LINE ( 'NONE', #40777, #15884 ) ;
#21906=DIRECTION ( 'NONE',  ( -1.000000000000000000, -0.000000000000000000, 0.000000000000000000 ) ) ;
#21910=DIRECTION ( 'NONE',  ( 0.000000000000000000, 0.000000000000000000, 1.000000000000000000 ) ) ;
#21927=CARTESIAN_POINT ( 'NONE',  ( -775.4999999999993179, -365.3551492539851893, -8.132432514707076621 ) ) ;
#21932=CARTESIAN_POINT ( 'NONE',  ( -775.4999999999993179, -512.9681489794448908, -339.9999999999999432 ) ) ;
#21942=EDGE_CURVE ( 'NONE', #2273, #3542, #10056, .T. ) ;
#21960=ORIENTED_EDGE ( 'NONE', *, *, #27442, .F. ) ;
#21961=CIRCLE ( 'NONE', #16784, 9.999999999999982236 ) ;
#21963=DIRECTION ( 'NONE',  ( -1.000000000000000000, -0.000000000000000000, -0.000000000000000000 ) ) ;
#22020=CARTESIAN_POINT ( 'NONE',  ( -773.4999999999993179, 26.27639943461401018, 900.0000000000001137 ) ) ;
#22025=CARTESIAN_POINT ( 'NONE',  ( 784.4999999999993179, -365.3551492539851893, -18.13243251470705886 ) ) ;
#22040=CARTESIAN_POINT ( 'NONE',  ( -784.4999999999993179, -544.8427095258973623, -369.9999999999999432 ) ) ;
#22048=FACE_BOUND ( 'NONE', #35186, .T. ) ;
#22058=EDGE_LOOP ( 'NONE', ( #16856, #45118, #43573, #30329 ) ) ;
#22107=ORIENTED_EDGE ( 'NONE', *, *, #20475, .F. ) ;
#22148=EDGE_CURVE ( 'NONE', #31022, #25758, #10496, .T. ) ;
#22178=EDGE_CURVE ( 'NONE', #16297, #32451, #38688, .T. ) ;
#22183=CARTESIAN_POINT ( 'NONE',  ( 786.4999999999993179, -513.1383975375929367, -349.9999999999999432 ) ) ;
#22191=CARTESIAN_POINT ( 'NONE',  ( -37.63011601220122770, -512.9681489794448908, -327.9999999999999432 ) ) ;
#22234=DIRECTION ( 'NONE',  ( 0.000000000000000000, 0.000000000000000000, 1.000000000000000000 ) ) ;
#22291=DIRECTION ( 'NONE',  ( -1.000000000000000000, -0.000000000000000000, 0.000000000000000000 ) ) ;
#22301=LINE ( 'NONE', #1064, #36465 ) ;
#22307=LINE ( 'NONE', #42883, #29181 ) ;
#22319=VERTEX_POINT ( 'NONE', #34294 ) ;
#22352=ORIENTED_EDGE ( 'NONE', *, *, #36529, .T. ) ;
#22374=ADVANCED_FACE ( 'NONE', ( #7728 ), #35434, .F. ) ;
#22384=DIRECTION ( 'NONE',  ( 0.000000000000000000, -0.3826834323650838421, -0.9238795325112891810 ) ) ;
#22405=ADVANCED_FACE ( 'NONE', ( #43056 ), #1012, .T. ) ;
#22408=EDGE_CURVE ( 'NONE', #757, #4454, #43286, .T. ) ;
#22426=ORIENTED_EDGE ( 'NONE', *, *, #30317, .F. ) ;
#22437=VERTEX_POINT ( 'NONE', #573 ) ;
#22484=FACE_OUTER_BOUND ( 'NONE', #45352, .T. ) ;
#22501=ADVANCED_FACE ( 'NONE', ( #42367 ), #39374, .T. ) ;
#22507=CARTESIAN_POINT ( 'NONE',  ( -26.63011601220122060, -365.3551492539851893, -18.13243251470705886 ) ) ;
#22515=DIRECTION ( 'NONE',  ( -1.000000000000000000, -0.000000000000000000, 0.000000000000000000 ) ) ;
#22547=VERTEX_POINT ( 'NONE', #25505 ) ;
#22553=ORIENTED_EDGE ( 'NONE', *, *, #15168, .T. ) ;
#22555=AXIS2_PLACEMENT_3D ( 'NONE', #28484, #10702, #18557 ) ;
#22592=VECTOR ( 'NONE', #44213, 1000.000000000000000 ) ;
#22615=EDGE_LOOP ( 'NONE', ( #34144, #15910, #5862, #39612 ) ) ;
#22643=DIRECTION ( 'NONE',  ( 0.000000000000000000, -0.3826834323650838421, -0.9238795325112891810 ) ) ;
#22653=VECTOR ( 'NONE', #4811, 1000.000000000000000 ) ;
#22663=DIRECTION ( 'NONE',  ( 0.000000000000000000, 0.6755902076156502511, 0.7372773368101330771 ) ) ;
#22668=VERTEX_POINT ( 'NONE', #30097 ) ;
#22673=VERTEX_POINT ( 'NONE', #40949 ) ;
#22681=DIRECTION ( 'NONE',  ( 1.000000000000000000, 0.000000000000000000, 0.000000000000000000 ) ) ;
#22682=DIRECTION ( 'NONE',  ( 1.000000000000000000, -0.000000000000000000, -0.000000000000000000 ) ) ;
#22727=ORIENTED_EDGE ( 'NONE', *, *, #17646, .T. ) ;
#22761=CARTESIAN_POINT ( 'NONE',  ( -26.63011601220122060, 26.27639943461401018, 900.0000000000001137 ) ) ;
#22771=ORIENTED_EDGE ( 'NONE', *, *, #21942, .F. ) ;
#22776=CARTESIAN_POINT ( 'NONE',  ( -28.63011601220122415, -513.1383975375929367, -369.9999999999999432 ) ) ;
#22800=LINE ( 'NONE', #33879, #7158 ) ;
#22806=EDGE_LOOP ( 'NONE', ( #36987, #15846, #26373, #28650, #19392, #40525, #30126, #40396, #28488, #26953, #1480, #7353 ) ) ;
#22832=ORIENTED_EDGE ( 'NONE', *, *, #24269, .F. ) ;
#22833=VERTEX_POINT ( 'NONE', #40289 ) ;
#22859=CARTESIAN_POINT ( 'NONE',  ( 773.4999999999993179, -494.6608068873671300, -357.6536686473015720 ) ) ;
#22914=CARTESIAN_POINT ( 'NONE',  ( -773.4999999999993179, 26.27639943461401018, 900.0000000000001137 ) ) ;
#22925=LINE ( 'NONE', #37017, #26236 ) ;
#22946=EDGE_CURVE ( 'NONE', #32451, #40161, #45572, .T. ) ;
#22956=DIRECTION ( 'NONE',  ( -1.000000000000000000, -0.000000000000000000, -0.000000000000000000 ) ) ;
#22973=DIRECTION ( 'NONE',  ( 0.000000000000000000, 0.000000000000000000, 1.000000000000000000 ) ) ;
#22978=CARTESIAN_POINT ( 'NONE',  ( -786.4999999999993179, -494.6608068873671300, -357.6536686473015720 ) ) ;
#23012=LINE ( 'NONE', #37106, #41806 ) ;
#23014=LINE ( 'NONE', #9169, #29319 ) ;
#23021=CIRCLE ( 'NONE', #34071, 9.999999999999982236 ) ;
#23036=CIRCLE ( 'NONE', #3143, 9.999999999999982236 ) ;
#23040=ORIENTED_EDGE ( 'NONE', *, *, #25157, .F. ) ;
#23065=ORIENTED_EDGE ( 'NONE', *, *, #5182, .F. ) ;
#23097=DIRECTION ( 'NONE',  ( 0.000000000000000000, 0.6755902076156502511, 0.7372773368101330771 ) ) ;
#23102=ORIENTED_EDGE ( 'NONE', *, *, #13502, .F. ) ;
#23127=( GEOMETRIC_REPRESENTATION_CONTEXT ( 3 ) GLOBAL_UNCERTAINTY_ASSIGNED_CONTEXT ( ( #6241 ) ) GLOBAL_UNIT_ASSIGNED_CONTEXT ( ( #45148, #3342, #38442 ) ) REPRESENTATION_CONTEXT ( 'NONE', 'WORKASPACE' ) );
#23153=CARTESIAN_POINT ( 'NONE',  ( 0.000000000000000000, 0.000000000000000000, 0.000000000000000000 ) ) ;
#23160=ORIENTED_EDGE ( 'NONE', *, *, #14545, .T. ) ;
#23170=CARTESIAN_POINT ( 'NONE',  ( -26.63011601220122060, -513.1383975375929367, -369.9999999999999432 ) ) ;
#23212=VERTEX_POINT ( 'NONE', #2451 ) ;
#23219=AXIS2_PLACEMENT_3D ( 'NONE', #28046, #6800, #34975 ) ;
#23222=EDGE_CURVE ( 'NONE', #2103, #32355, #38033, .T. ) ;
#23251=VERTEX_POINT ( 'NONE', #23912 ) ;
#23258=AXIS2_PLACEMENT_3D ( 'NONE', #10736, #4275, #18367 ) ;
#23265=EDGE_CURVE ( 'NONE', #24190, #36920, #45421, .T. ) ;
#23270=ORIENTED_EDGE ( 'NONE', *, *, #1487, .F. ) ;
#23277=AXIS2_PLACEMENT_3D ( 'NONE', #12179, #16318, #8726 ) ;
#23300=EDGE_CURVE ( 'NONE', #22833, #30278, #41749, .T. ) ;
#23320=EDGE_CURVE ( 'NONE', #12731, #37281, #13545, .T. ) ;
#23360=ORIENTED_EDGE ( 'NONE', *, *, #4428, .T. ) ;
#23364=CARTESIAN_POINT ( 'NONE',  ( -786.4999999999993179, -563.3203001761230553, -342.3463313526983143 ) ) ;
#23376=LINE ( 'NONE', #16012, #41656 ) ;
#23382=AXIS2_PLACEMENT_3D ( 'NONE', #10066, #31539, #24357 ) ;
#23393=ORIENTED_EDGE ( 'NONE', *, *, #3799, .F. ) ;
#23406=DIRECTION ( 'NONE',  ( -1.000000000000000000, -0.000000000000000000, 0.000000000000000000 ) ) ;
#23425=FACE_OUTER_BOUND ( 'NONE', #43616, .T. ) ;
#23428=CARTESIAN_POINT ( 'NONE',  ( -786.4999999999993179, -512.9681489794448908, -329.9999999999999432 ) ) ;
#23481=VECTOR ( 'NONE', #34912, 1000.000000000000000 ) ;
#23504=ADVANCED_FACE ( 'NONE', ( #10520, #24595, #21155 ), #10999, .F. ) ;
#23506=VERTEX_POINT ( 'NONE', #4297 ) ;
#23552=CARTESIAN_POINT ( 'NONE',  ( 786.4999999999993179, -563.3203001761230553, -342.3463313526983143 ) ) ;
#23553=EDGE_CURVE ( 'NONE', #19003, #21254, #25520, .T. ) ;
#23562=ORIENTED_EDGE ( 'NONE', *, *, #7983, .T. ) ;
#23580=ADVANCED_FACE ( 'NONE', ( #14917 ), #32693, .F. ) ;
#23621=ORIENTED_EDGE ( 'NONE', *, *, #21836, .T. ) ;
#23649=LINE ( 'NONE', #20431, #32765 ) ;
#23667=LINE ( 'NONE', #9142, #258 ) ;
#23692=CARTESIAN_POINT ( 'NONE',  ( 775.4999999999993179, -355.4967352946684969, -16.45562775363632113 ) ) ;
#23699=ORIENTED_EDGE ( 'NONE', *, *, #32627, .F. ) ;
#23706=CARTESIAN_POINT ( 'NONE',  ( -784.4999999999993179, -513.1383975375929367, -367.9999999999999432 ) ) ;
#23715=CARTESIAN_POINT ( 'NONE',  ( 784.4999999999993179, -857.0166862835568509, -63.94525337997358605 ) ) ;
#23717=EDGE_LOOP ( 'NONE', ( #4226, #41991, #17970, #4186 ) ) ;
#23722=ORIENTED_EDGE ( 'NONE', *, *, #19325, .F. ) ;
#23727=ORIENTED_EDGE ( 'NONE', *, *, #23300, .T. ) ;
#23743=CARTESIAN_POINT ( 'NONE',  ( -28.63011601220122415, -512.9681489794448908, -327.9999999999999432 ) ) ;
#23827=EDGE_CURVE ( 'NONE', #7478, #1429, #25530, .T. ) ;
#23841=EDGE_CURVE ( 'NONE', #39212, #40621, #33585, .T. ) ;
#23853=CARTESIAN_POINT ( 'NONE',  ( 786.4999999999993179, -436.2161768796786987, 399.7184814855371542 ) ) ;
#23854=ORIENTED_EDGE ( 'NONE', *, *, #3799, .T. ) ;
#23904=EDGE_CURVE ( 'NONE', #7856, #33261, #35102, .T. ) ;
#23912=CARTESIAN_POINT ( 'NONE',  ( 773.4999999999993179, -512.9681489794448908, -350.0000000000000000 ) ) ;
#23924=FACE_OUTER_BOUND ( 'NONE', #415, .T. ) ;
#23973=DIRECTION ( 'NONE',  ( -0.000000000000000000, -0.000000000000000000, -1.000000000000000000 ) ) ;
#23990=CARTESIAN_POINT ( 'NONE',  ( 1007.605605532488426, 262.9227088301245203, 634.7515695135432452 ) ) ;
#23991=VECTOR ( 'NONE', #16956, 1000.000000000000000 ) ;
#23997=LINE ( 'NONE', #35089, #38308 ) ;
#24030=AXIS2_PLACEMENT_3D ( 'NONE', #33319, #12530, #1895 ) ;
#24061=AXIS2_PLACEMENT_3D ( 'NONE', #43697, #22681, #2118 ) ;
#24084=ORIENTED_EDGE ( 'NONE', *, *, #21315, .F. ) ;
#24102=CARTESIAN_POINT ( 'NONE',  ( 773.4999999999993179, -563.3203001761230553, -342.3463313526983143 ) ) ;
#24114=VECTOR ( 'NONE', #27966, 1000.000000000000000 ) ;
#24127=CARTESIAN_POINT ( 'NONE',  ( -37.63011601220122770, -359.5698779088871788, -26.28906389436296109 ) ) ;
#24165=EDGE_CURVE ( 'NONE', #34816, #7404, #31655, .T. ) ;
#24174=CARTESIAN_POINT ( 'NONE',  ( 786.4999999999993179, -512.9681489794448908, -339.9999999999999432 ) ) ;
#24184=AXIS2_PLACEMENT_3D ( 'NONE', #27105, #31245, #13015 ) ;
#24190=VERTEX_POINT ( 'NONE', #37735 ) ;
#24244=AXIS2_PLACEMENT_3D ( 'NONE', #44868, #34215, #2590 ) ;
#24245=ORIENTED_EDGE ( 'NONE', *, *, #14278, .F. ) ;
#24264=CARTESIAN_POINT ( 'NONE',  ( 784.4999999999993179, -512.9681489794448908, -327.9999999999999432 ) ) ;
#24269=EDGE_CURVE ( 'NONE', #5117, #518, #5867, .T. ) ;
#24270=PLANE ( 'NONE',  #3337 ) ;
#24283=DIRECTION ( 'NONE',  ( 1.000000000000000000, 0.000000000000000000, -0.000000000000000000 ) ) ;
#24295=CARTESIAN_POINT ( 'NONE',  ( -28.63011601220122415, -512.9681489794448908, -339.9999999999999432 ) ) ;
#24304=CARTESIAN_POINT ( 'NONE',  ( -775.4999999999993179, -110.5936016518799221, 750.6326042729449455 ) ) ;
#24319=FACE_OUTER_BOUND ( 'NONE', #19320, .T. ) ;
#24320=ADVANCED_FACE ( 'NONE', ( #37508 ), #42519, .T. ) ;
#24322=VERTEX_POINT ( 'NONE', #14114 ) ;
#24325=CARTESIAN_POINT ( 'NONE',  ( -26.63011601220122060, -544.8427095258973623, -350.0000000000000000 ) ) ;
#24328=DIRECTION ( 'NONE',  ( 1.000000000000000000, -0.000000000000000000, -0.000000000000000000 ) ) ;
#24339=DIRECTION ( 'NONE',  ( 0.000000000000000000, 0.000000000000000000, 1.000000000000000000 ) ) ;
#24353=ORIENTED_EDGE ( 'NONE', *, *, #30000, .F. ) ;
#24357=DIRECTION ( 'NONE',  ( 0.000000000000000000, 0.000000000000000000, 1.000000000000000000 ) ) ;
#24365=ADVANCED_FACE ( 'NONE', ( #42280, #41210 ), #10885, .F. ) ;
#24418=VERTEX_POINT ( 'NONE', #36048 ) ;
#24423=EDGE_CURVE ( 'NONE', #30803, #34298, #15264, .T. ) ;
#24441=ORIENTED_EDGE ( 'NONE', *, *, #22148, .T. ) ;
#24493=CARTESIAN_POINT ( 'NONE',  ( -26.63011601220122060, -563.3203001761230553, -342.3463313526983143 ) ) ;
#24497=CARTESIAN_POINT ( 'NONE',  ( -26.63011601220122060, -512.9681489794448908, -339.9999999999999432 ) ) ;
#24505=DIRECTION ( 'NONE',  ( 0.000000000000000000, 0.000000000000000000, 1.000000000000000000 ) ) ;
#24544=CARTESIAN_POINT ( 'NONE',  ( 775.4999999999993179, -512.9681489794448908, -327.9999999999999432 ) ) ;
#24553=FACE_OUTER_BOUND ( 'NONE', #9436, .T. ) ;
#24595=FACE_OUTER_BOUND ( 'NONE', #29701, .T. ) ;
#24604=AXIS2_PLACEMENT_3D ( 'NONE', #26598, #9053, #11851 ) ;
#24626=VECTOR ( 'NONE', #29632, 1000.000000000000000 ) ;
#24646=EDGE_CURVE ( 'NONE', #2495, #17065, #1159, .T. ) ;
#24650=PRODUCT_CONTEXT ( 'NONE', #27853, 'mechanical' ) ;
#24739=AXIS2_PLACEMENT_3D ( 'NONE', #4073, #29009, #35937 ) ;
#24745=AXIS2_PLACEMENT_3D ( 'NONE', #42832, #39155, #11656 ) ;
#24761=ORIENTED_EDGE ( 'NONE', *, *, #15930, .T. ) ;
#24773=EDGE_LOOP ( 'NONE', ( #42516, #11216, #3726, #23722, #9788, #1259, #8720, #31880 ) ) ;
#24774=VECTOR ( 'NONE', #11687, 1000.000000000000000 ) ;
#24794=LINE ( 'NONE', #11172, #16515 ) ;
#24832=ORIENTED_EDGE ( 'NONE', *, *, #40181, .F. ) ;
#24860=CARTESIAN_POINT ( 'NONE',  ( -786.4999999999993179, -512.9681489794448908, -339.9999999999999432 ) ) ;
#24867=FACE_OUTER_BOUND ( 'NONE', #40369, .T. ) ;
#24876=VECTOR ( 'NONE', #30650, 1000.000000000000000 ) ;
#24878=DIRECTION ( 'NONE',  ( 1.000000000000000000, 0.000000000000000000, 0.000000000000000000 ) ) ;
#24886=EDGE_LOOP ( 'NONE', ( #43134, #45083, #43472, #37265 ) ) ;
#24888=EDGE_LOOP ( 'NONE', ( #1640, #6553, #7564, #30756 ) ) ;
#24901=CARTESIAN_POINT ( 'NONE',  ( -786.4999999999993179, -512.9681489794448908, -339.9999999999999432 ) ) ;
#24914=FACE_OUTER_BOUND ( 'NONE', #28343, .T. ) ;
#24932=ORIENTED_EDGE ( 'NONE', *, *, #11519, .F. ) ;
#24952=DIRECTION ( 'NONE',  ( 0.000000000000000000, 0.000000000000000000, 1.000000000000000000 ) ) ;
#24955=EDGE_CURVE ( 'NONE', #1029, #37198, #21864, .T. ) ;
#24966=DIRECTION ( 'NONE',  ( 1.000000000000000000, -0.000000000000000000, -0.000000000000000000 ) ) ;
#25001=ORIENTED_EDGE ( 'NONE', *, *, #43293, .F. ) ;
#25025=LINE ( 'NONE', #21335, #35695 ) ;
#25029=LINE ( 'NONE', #18117, #34252 ) ;
#25069=ORIENTED_EDGE ( 'NONE', *, *, #20475, .T. ) ;
#25096=LINE ( 'NONE', #14732, #21751 ) ;
#25100=CARTESIAN_POINT ( 'NONE',  ( 775.4999999999993179, -512.9681489794448908, -339.9999999999999432 ) ) ;
#25157=EDGE_CURVE ( 'NONE', #16297, #30803, #15250, .T. ) ;
#25162=CARTESIAN_POINT ( 'NONE',  ( -775.4999999999993179, -513.1383975375929367, -350.0000000000000000 ) ) ;
#25216=ORIENTED_EDGE ( 'NONE', *, *, #2708, .T. ) ;
#25229=EDGE_CURVE ( 'NONE', #10285, #32281, #38781, .T. ) ;
#25238=DIRECTION ( 'NONE',  ( 1.000000000000000000, -0.000000000000000000, -0.000000000000000000 ) ) ;
#25240=ORIENTED_EDGE ( 'NONE', *, *, #28330, .F. ) ;
#25275=FACE_OUTER_BOUND ( 'NONE', #39470, .T. ) ;
#25301=CARTESIAN_POINT ( 'NONE',  ( -28.63011601220122415, -365.3551492539851893, -18.13243251470705886 ) ) ;
#25302=LINE ( 'NONE', #32703, #39547 ) ;
#25304=FACE_OUTER_BOUND ( 'NONE', #37029, .T. ) ;
#25307=CARTESIAN_POINT ( 'NONE',  ( -786.4999999999993179, -110.5936016518799221, 750.6326042729449455 ) ) ;
#25339=ORIENTED_EDGE ( 'NONE', *, *, #19836, .T. ) ;
#25343=AXIS2_PLACEMENT_3D ( 'NONE', #2902, #28276, #38697 ) ;
#25352=FACE_OUTER_BOUND ( 'NONE', #16116, .T. ) ;
#25354=PLANE ( 'NONE',  #5538 ) ;
#25364=ORIENTED_EDGE ( 'NONE', *, *, #12787, .T. ) ;
#25380=CARTESIAN_POINT ( 'NONE',  ( -28.63011601220122415, -365.3551492539851893, -28.13243251470704109 ) ) ;
#25396=AXIS2_PLACEMENT_3D ( 'NONE', #38166, #2824, #38862 ) ;
#25449=VECTOR ( 'NONE', #26237, 1000.000000000000227 ) ;
#25455=ORIENTED_EDGE ( 'NONE', *, *, #22148, .F. ) ;
#25475=CARTESIAN_POINT ( 'NONE',  ( 786.4999999999993179, -513.1383975375929367, -349.9999999999999432 ) ) ;
#25485=EDGE_CURVE ( 'NONE', #37198, #1029, #9367, .T. ) ;
#25505=CARTESIAN_POINT ( 'NONE',  ( -37.63011601220122770, 22.32581219114657856, 895.6886905569881492 ) ) ;
#25520=CIRCLE ( 'NONE', #10023, 18.00000000000001421 ) ;
#25524=ORIENTED_EDGE ( 'NONE', *, *, #11876, .F. ) ;
#25530=LINE ( 'NONE', #21833, #1893 ) ;
#25536=DIRECTION ( 'NONE',  ( 1.000000000000000000, -0.000000000000000000, -0.000000000000000000 ) ) ;
#25539=AXIS2_PLACEMENT_3D ( 'NONE', #43743, #19489, #8672 ) ;
#25559=PLANE ( 'NONE',  #13152 ) ;
#25568=EDGE_LOOP ( 'NONE', ( #26316, #43174, #37220, #19597 ) ) ;
#25584=EDGE_LOOP ( 'NONE', ( #5564, #41302, #23040, #33348, #2041, #38945, #6260, #23699, #3293, #44366, #2247 ) ) ;
#25591=AXIS2_PLACEMENT_3D ( 'NONE', #17237, #31323, #27870 ) ;
#25602=CARTESIAN_POINT ( 'NONE',  ( -784.4999999999993179, -513.1383975375929367, -369.9999999999999432 ) ) ;
#25609=ORIENTED_EDGE ( 'NONE', *, *, #28130, .T. ) ;
#25617=FACE_OUTER_BOUND ( 'NONE', #23717, .T. ) ;
#25629=DIRECTION ( 'NONE',  ( 1.000000000000000000, -0.000000000000000000, -0.000000000000000000 ) ) ;
#25655=EDGE_LOOP ( 'NONE', ( #7798, #33639, #1734, #37379, #32566, #22727 ) ) ;
#25661=FACE_OUTER_BOUND ( 'NONE', #42443, .T. ) ;
#25731=DIRECTION ( 'NONE',  ( -1.000000000000000000, -0.000000000000000000, -0.000000000000000000 ) ) ;
#25735=ORIENTED_EDGE ( 'NONE', *, *, #43262, .T. ) ;
#25739=FACE_BOUND ( 'NONE', #31660, .T. ) ;
#25741=ORIENTED_EDGE ( 'NONE', *, *, #13502, .T. ) ;
#25756=CARTESIAN_POINT ( 'NONE',  ( 775.4999999999993179, -513.1383975375929367, -349.9999999999999432 ) ) ;
#25758=VERTEX_POINT ( 'NONE', #25602 ) ;
#25760=CARTESIAN_POINT ( 'NONE',  ( 786.4999999999993179, -513.1383975375929367, -369.9999999999999432 ) ) ;
#25769=FACE_BOUND ( 'NONE', #45695, .T. ) ;
#25780=PLANE ( 'NONE',  #4326 ) ;
#25795=EDGE_CURVE ( 'NONE', #69, #27963, #27070, .T. ) ;
#25814=CARTESIAN_POINT ( 'NONE',  ( -26.63011601220122060, 22.32581219114657856, 895.6886905569881492 ) ) ;
#25830=ORIENTED_EDGE ( 'NONE', *, *, #12787, .F. ) ;
#25851=LINE ( 'NONE', #35554, #19496 ) ;
#25879=CARTESIAN_POINT ( 'NONE',  ( -28.63011601220122415, -355.4967352946684969, -16.45562775363623587 ) ) ;
#25954=VERTEX_POINT ( 'NONE', #30407 ) ;
#25972=LINE ( 'NONE', #16270, #42573 ) ;
#26022=PLANE ( 'NONE',  #36130 ) ;
#26026=DIRECTION ( 'NONE',  ( 0.000000000000000000, 0.000000000000000000, 1.000000000000000000 ) ) ;
#26103=CARTESIAN_POINT ( 'NONE',  ( -37.63011601220122770, -563.3203001761231690, -342.3463313526983143 ) ) ;
#26109=CIRCLE ( 'NONE', #4006, 20.00000000000001776 ) ;
#26110=AXIS2_PLACEMENT_3D ( 'NONE', #13054, #9120, #8899 ) ;
#26125=FACE_OUTER_BOUND ( 'NONE', #21038, .T. ) ;
#26139=VERTEX_POINT ( 'NONE', #19558 ) ;
#26171=VECTOR ( 'NONE', #6119, 1000.000000000000000 ) ;
#26236=VECTOR ( 'NONE', #5372, 1000.000000000000000 ) ;
#26237=DIRECTION ( 'NONE',  ( 0.000000000000000000, 0.3826834323650836200, 0.9238795325112892920 ) ) ;
#26242=AXIS2_PLACEMENT_3D ( 'NONE', #598, #11680, #3616 ) ;
#26262=FACE_OUTER_BOUND ( 'NONE', #42893, .T. ) ;
#26293=VECTOR ( 'NONE', #661, 1000.000000000000000 ) ;
#26305=ADVANCED_FACE ( 'NONE', ( #2700 ), #3146, .F. ) ;
#26316=ORIENTED_EDGE ( 'NONE', *, *, #45039, .F. ) ;
#26327=ORIENTED_EDGE ( 'NONE', *, *, #35742, .F. ) ;
#26350=AXIS2_PLACEMENT_3D ( 'NONE', #12808, #37526, #37756 ) ;
#26363=AXIS2_PLACEMENT_3D ( 'NONE', #12553, #30106, #33340 ) ;
#26373=ORIENTED_EDGE ( 'NONE', *, *, #29702, .T. ) ;
#26400=DIRECTION ( 'NONE',  ( 1.000000000000000000, 0.000000000000000000, 0.000000000000000000 ) ) ;
#26415=ORIENTED_EDGE ( 'NONE', *, *, #33987, .F. ) ;
#26431=CARTESIAN_POINT ( 'NONE',  ( -66.63011601220125613, -365.3551492539851893, -8.132432514707076621 ) ) ;
#26462=EDGE_CURVE ( 'NONE', #2273, #22437, #45512, .T. ) ;
#26498=CARTESIAN_POINT ( 'NONE',  ( -786.4999999999993179, -512.9681489794448908, -327.9999999999999432 ) ) ;
#26560=DIRECTION ( 'NONE',  ( 0.000000000000000000, 1.000000000000000000, 0.000000000000000000 ) ) ;
#26575=LINE ( 'NONE', #37441, #19737 ) ;
#26595=VERTEX_POINT ( 'NONE', #23692 ) ;
#26598=CARTESIAN_POINT ( 'NONE',  ( -784.4999999999993179, -513.1383975375929367, -349.9999999999999432 ) ) ;
#26604=FACE_OUTER_BOUND ( 'NONE', #32726, .T. ) ;
#26644=CYLINDRICAL_SURFACE ( 'NONE', #15937, 10.00000000000000888 ) ;
#26645=ORIENTED_EDGE ( 'NONE', *, *, #11519, .T. ) ;
#26675=CARTESIAN_POINT ( 'NONE',  ( -784.4999999999993179, -365.3551492539851893, -8.132432514707076621 ) ) ;
#26690=ORIENTED_EDGE ( 'NONE', *, *, #17347, .T. ) ;
#26711=CARTESIAN_POINT ( 'NONE',  ( -39.63011601220123481, -512.9681489794448908, -339.9999999999999432 ) ) ;
#26715=DIRECTION ( 'NONE',  ( 0.000000000000000000, 0.3826834323650836756, 0.9238795325112892920 ) ) ;
#26727=EDGE_LOOP ( 'NONE', ( #28147, #40293, #45415, #19312, #31689, #28170, #8718, #23270, #13934, #18842, #4607 ) ) ;
#26758=ORIENTED_EDGE ( 'NONE', *, *, #12516, .T. ) ;
#26761=CARTESIAN_POINT ( 'NONE',  ( -26.63011601220122060, -512.9681489794448908, -327.9999999999999432 ) ) ;
#26764=ORIENTED_EDGE ( 'NONE', *, *, #28389, .F. ) ;
#26772=PLANE ( 'NONE',  #11481 ) ;
#26796=AXIS2_PLACEMENT_3D ( 'NONE', #39543, #10478, #13737 ) ;
#26825=DIRECTION ( 'NONE',  ( 0.000000000000000000, 0.000000000000000000, 1.000000000000000000 ) ) ;
#26856=AXIS2_PLACEMENT_3D ( 'NONE', #25475, #36555, #1440 ) ;
#26858=AXIS2_PLACEMENT_3D ( 'NONE', #23153, #34241, #6075 ) ;
#26888=VECTOR ( 'NONE', #29200, 1000.000000000000114 ) ;
#26936=EDGE_CURVE ( 'NONE', #29224, #39697, #1996, .T. ) ;
#26945=CARTESIAN_POINT ( 'NONE',  ( -37.63011601220122770, -110.5936016518799221, 750.6326042729449455 ) ) ;
#26953=ORIENTED_EDGE ( 'NONE', *, *, #36529, .F. ) ;
#26985=EDGE_CURVE ( 'NONE', #19341, #45642, #25972, .T. ) ;
#26993=AXIS2_PLACEMENT_3D ( 'NONE', #27618, #41489, #34559 ) ;
#27003=ORIENTED_EDGE ( 'NONE', *, *, #24646, .F. ) ;
#27029=CARTESIAN_POINT ( 'NONE',  ( -775.4999999999993179, -365.3551492539851893, -28.13243251470704109 ) ) ;
#27061=VECTOR ( 'NONE', #19795, 999.9999999999998863 ) ;
#27070=CIRCLE ( 'NONE', #41084, 19.99999999999990763 ) ;
#27079=CARTESIAN_POINT ( 'NONE',  ( -784.4999999999993179, -857.0166862835568509, -63.94525337997358605 ) ) ;
#27105=CARTESIAN_POINT ( 'NONE',  ( -786.4999999999993179, -110.5936016518799221, 750.6326042729449455 ) ) ;
#27106=ORIENTED_EDGE ( 'NONE', *, *, #7243, .T. ) ;
#27124=DIRECTION ( 'NONE',  ( 0.000000000000000000, 0.000000000000000000, 1.000000000000000000 ) ) ;
#27142=CARTESIAN_POINT ( 'NONE',  ( 786.4999999999993179, -512.9681489794448908, -350.0000000000000000 ) ) ;
#27178=CARTESIAN_POINT ( 'NONE',  ( -784.4999999999993179, -563.3203001761231690, -342.3463313526983143 ) ) ;
#27198=FACE_OUTER_BOUND ( 'NONE', #41886, .T. ) ;
#27232=ORIENTED_EDGE ( 'NONE', *, *, #18259, .F. ) ;
#27292=CARTESIAN_POINT ( 'NONE',  ( -786.4999999999993179, -434.0043448692482002, 397.6917108626901154 ) ) ;
#27389=ORIENTED_EDGE ( 'NONE', *, *, #24423, .T. ) ;
#27417=CARTESIAN_POINT ( 'NONE',  ( 775.4999999999993179, -513.1383975375929367, -350.0000000000000000 ) ) ;
#27437=ORIENTED_EDGE ( 'NONE', *, *, #28592, .F. ) ;
#27442=EDGE_CURVE ( 'NONE', #30488, #14297, #27809, .T. ) ;
#27486=PRODUCT_DEFINITION_CONTEXT ( 'detailed design', #37001, 'design' ) ;
#27509=ORIENTED_EDGE ( 'NONE', *, *, #34612, .F. ) ;
#27518=CARTESIAN_POINT ( 'NONE',  ( -39.63011601220123481, -365.3551492539851893, -18.13243251470705886 ) ) ;
#27521=EDGE_CURVE ( 'NONE', #24322, #27963, #31038, .T. ) ;
#27547=AXIS2_PLACEMENT_3D ( 'NONE', #25100, #14953, #43564 ) ;
#27555=ORIENTED_EDGE ( 'NONE', *, *, #15681, .T. ) ;
#27560=CYLINDRICAL_SURFACE ( 'NONE', #40288, 19.99999999999990763 ) ;
#27565=DIRECTION ( 'NONE',  ( 0.000000000000000000, 0.000000000000000000, 1.000000000000000000 ) ) ;
#27569=MECHANICAL_DESIGN_GEOMETRIC_PRESENTATION_REPRESENTATION('',(#18746),#23127);
#27575=FACE_OUTER_BOUND ( 'NONE', #27719, .T. ) ;
#27618=CARTESIAN_POINT ( 'NONE',  ( -37.63011601220122770, -365.3551492539851893, -18.13243251470705886 ) ) ;
#27641=FACE_OUTER_BOUND ( 'NONE', #19477, .T. ) ;
#27658=DIRECTION ( 'NONE',  ( 0.000000000000000000, 0.000000000000000000, -1.000000000000000000 ) ) ;
#27669=ORIENTED_EDGE ( 'NONE', *, *, #37429, .T. ) ;
#27672=VECTOR ( 'NONE', #42296, 1000.000000000000000 ) ;
#27685=CARTESIAN_POINT ( 'NONE',  ( -28.63011601220122415, -513.1383975375929367, -349.9999999999999432 ) ) ;
#27687=CARTESIAN_POINT ( 'NONE',  ( 786.4999999999993179, -512.9681489794448908, -350.0000000000000000 ) ) ;
#27719=EDGE_LOOP ( 'NONE', ( #42618, #37782, #43725, #2507 ) ) ;
#27744=EDGE_CURVE ( 'NONE', #7984, #35816, #24794, .T. ) ;
#27759=DIRECTION ( 'NONE',  ( -1.000000000000000000, -0.000000000000000000, -0.000000000000000000 ) ) ;
#27773=ORIENTED_EDGE ( 'NONE', *, *, #7148, .T. ) ;
#27791=EDGE_LOOP ( 'NONE', ( #17806, #25741, #44292, #11488 ) ) ;
#27806=EDGE_CURVE ( 'NONE', #2064, #7404, #32191, .T. ) ;
#27809=LINE ( 'NONE', #45370, #37908 ) ;
#27817=CARTESIAN_POINT ( 'NONE',  ( 1007.605605532488426, 323.4107432173689176, 352.9408934102648345 ) ) ;
#27821=LINE ( 'NONE', #41230, #1033 ) ;
#27853=APPLICATION_CONTEXT ( 'automotive_design' ) ;
#27870=DIRECTION ( 'NONE',  ( 0.000000000000000000, 0.000000000000000000, 1.000000000000000000 ) ) ;
#27876=DIRECTION ( 'NONE',  ( 0.000000000000000000, 0.000000000000000000, 1.000000000000000000 ) ) ;
#27884=CARTESIAN_POINT ( 'NONE',  ( -775.4999999999993179, -365.3551492539851893, -18.13243251470705886 ) ) ;
#27921=DIRECTION ( 'NONE',  ( -1.000000000000000000, -0.000000000000000000, -0.000000000000000000 ) ) ;
#27963=VERTEX_POINT ( 'NONE', #10954 ) ;
#27966=DIRECTION ( 'NONE',  ( -1.000000000000000000, -0.000000000000000000, -0.000000000000000000 ) ) ;
#27973=CIRCLE ( 'NONE', #45674, 20.00000000000001776 ) ;
#27976=CARTESIAN_POINT ( 'NONE',  ( 773.4999999999993179, -512.9681489794448908, -329.9999999999999432 ) ) ;
#27982=CARTESIAN_POINT ( 'NONE',  ( -26.63011601220122060, -365.3551492539851893, -28.13243251470704109 ) ) ;
#28006=DIRECTION ( 'NONE',  ( 0.000000000000000000, 0.7372773368101328550, -0.6755902076156506952 ) ) ;
#28009=ORIENTED_EDGE ( 'NONE', *, *, #41026, .F. ) ;
#28022=EDGE_LOOP ( 'NONE', ( #12619, #2615, #28778, #18344 ) ) ;
#28033=DIRECTION ( 'NONE',  ( 0.000000000000000000, 0.000000000000000000, 1.000000000000000000 ) ) ;
#28046=CARTESIAN_POINT ( 'NONE',  ( 784.4999999999993179, -512.9681489794448908, -339.9999999999999432 ) ) ;
#28049=EDGE_CURVE ( 'NONE', #37811, #8747, #25025, .T. ) ;
#28053=ADVANCED_FACE ( 'NONE', ( #312 ), #40487, .F. ) ;
#28068=ORIENTED_EDGE ( 'NONE', *, *, #45051, .T. ) ;
#28077=EDGE_CURVE ( 'NONE', #32451, #34298, #29082, .T. ) ;
#28088=LINE ( 'NONE', #14239, #33744 ) ;
#28090=EDGE_CURVE ( 'NONE', #39064, #42371, #33540, .T. ) ;
#28100=DIRECTION ( 'NONE',  ( -1.000000000000000000, -0.000000000000000000, -0.000000000000000000 ) ) ;
#28130=EDGE_CURVE ( 'NONE', #30797, #44478, #41602, .T. ) ;
#28147=ORIENTED_EDGE ( 'NONE', *, *, #15051, .F. ) ;
#28170=ORIENTED_EDGE ( 'NONE', *, *, #15926, .F. ) ;
#28235=ORIENTED_EDGE ( 'NONE', *, *, #5817, .T. ) ;
#28267=DIRECTION ( 'NONE',  ( 0.000000000000000000, 0.000000000000000000, 1.000000000000000000 ) ) ;
#28276=DIRECTION ( 'NONE',  ( 0.000000000000000000, -0.9238795325112892920, 0.3826834323650836756 ) ) ;
#28294=DIRECTION ( 'NONE',  ( 1.000000000000000000, 0.000000000000000000, -0.000000000000000000 ) ) ;
#28309=DIRECTION ( 'NONE',  ( 0.000000000000000000, 0.000000000000000000, 1.000000000000000000 ) ) ;
#28327=LINE ( 'NONE', #23715, #30579 ) ;
#28330=EDGE_CURVE ( 'NONE', #36107, #19341, #3219, .T. ) ;
#28343=EDGE_LOOP ( 'NONE', ( #39183, #19208, #42641, #42631, #27106, #968, #18774, #24441, #29229, #5874, #40794 ) ) ;
#28389=EDGE_CURVE ( 'NONE', #34942, #10012, #25851, .T. ) ;
#28399=VERTEX_POINT ( 'NONE', #39959 ) ;
#28484=CARTESIAN_POINT ( 'NONE',  ( 746.4999999999993179, -365.3551492539851893, -18.13243251470705886 ) ) ;
#28488=ORIENTED_EDGE ( 'NONE', *, *, #33660, .F. ) ;
#28549=CYLINDRICAL_SURFACE ( 'NONE', #8574, 9.999999999999980460 ) ;
#28583=VECTOR ( 'NONE', #2932, 1000.000000000000000 ) ;
#28592=EDGE_CURVE ( 'NONE', #19341, #25954, #11555, .T. ) ;
#28613=CARTESIAN_POINT ( 'NONE',  ( 786.4999999999993179, -30.07539427629363260, 756.1153575698150462 ) ) ;
#28649=CARTESIAN_POINT ( 'NONE',  ( -28.63011601220122415, 22.32581219114657856, 895.6886905569881492 ) ) ;
#28650=ORIENTED_EDGE ( 'NONE', *, *, #38277, .F. ) ;
#28665=EDGE_CURVE ( 'NONE', #21254, #17123, #37143, .T. ) ;
#28704=PLANE ( 'NONE',  #5012 ) ;
#28778=ORIENTED_EDGE ( 'NONE', *, *, #4722, .T. ) ;
#28800=CARTESIAN_POINT ( 'NONE',  ( 786.4999999999993179, -544.8427095258973623, -350.0000000000000000 ) ) ;
#28805=CARTESIAN_POINT ( 'NONE',  ( -26.63011601220122060, -110.5936016518799221, 750.6326042729449455 ) ) ;
#28841=ORIENTED_EDGE ( 'NONE', *, *, #317, .F. ) ;
#28850=CARTESIAN_POINT ( 'NONE',  ( -786.4999999999993179, -512.9681489794448908, -339.9999999999999432 ) ) ;
#28863=ORIENTED_EDGE ( 'NONE', *, *, #12245, .F. ) ;
#28895=CYLINDRICAL_SURFACE ( 'NONE', #10598, 18.00000000000001421 ) ;
#28919=AXIS2_PLACEMENT_3D ( 'NONE', #2716, #34348, #34583 ) ;
#28929=CARTESIAN_POINT ( 'NONE',  ( -26.63011601220122060, -513.1383975375929367, -369.9999999999999432 ) ) ;
#28930=ORIENTED_EDGE ( 'NONE', *, *, #23320, .T. ) ;
#28968=CARTESIAN_POINT ( 'NONE',  ( 779.9999999999993179, -513.1383975375929367, -367.9999999999999432 ) ) ;
#29009=DIRECTION ( 'NONE',  ( 1.000000000000000000, -0.000000000000000000, -0.000000000000000000 ) ) ;
#29011=CARTESIAN_POINT ( 'NONE',  ( 786.4999999999993179, -496.5085659523897448, -356.8883017825714319 ) ) ;
#29013=DIRECTION ( 'NONE',  ( 0.000000000000000000, 0.000000000000000000, 1.000000000000000000 ) ) ;
#29030=CARTESIAN_POINT ( 'NONE',  ( -37.63011601220122770, -355.4967352946684969, -16.45562775363632113 ) ) ;
#29061=CARTESIAN_POINT ( 'NONE',  ( -784.4999999999993179, -355.4967352946684969, -16.45562775363623587 ) ) ;
#29082=CIRCLE ( 'NONE', #17268, 18.00000000000001421 ) ;
#29111=ORIENTED_EDGE ( 'NONE', *, *, #1776, .F. ) ;
#29168=ORIENTED_EDGE ( 'NONE', *, *, #29862, .T. ) ;
#29181=VECTOR ( 'NONE', #36404, 1000.000000000000000 ) ;
#29198=EDGE_CURVE ( 'NONE', #39517, #6318, #12846, .T. ) ;
#29200=DIRECTION ( 'NONE',  ( 0.000000000000000000, -0.6755902076156505842, -0.7372773368101328550 ) ) ;
#29206=CIRCLE ( 'NONE', #30646, 19.99999999999990763 ) ;
#29222=EDGE_CURVE ( 'NONE', #40010, #33295, #33518, .T. ) ;
#29224=VERTEX_POINT ( 'NONE', #25380 ) ;
#29229=ORIENTED_EDGE ( 'NONE', *, *, #12516, .F. ) ;
#29240=CARTESIAN_POINT ( 'NONE',  ( -28.63011601220122415, -512.9681489794448908, -352.0000000000000000 ) ) ;
#29316=DIRECTION ( 'NONE',  ( 1.000000000000000000, 0.000000000000000000, 0.000000000000000000 ) ) ;
#29319=VECTOR ( 'NONE', #16567, 1000.000000000000000 ) ;
#29351=EDGE_LOOP ( 'NONE', ( #39002, #35405, #12879, #30845, #37954, #34340 ) ) ;
#29355=DIRECTION ( 'NONE',  ( 0.000000000000000000, 0.000000000000000000, -1.000000000000000000 ) ) ;
#29374=DIRECTION ( 'NONE',  ( 0.000000000000000000, 0.000000000000000000, 1.000000000000000000 ) ) ;
#29390=ORIENTED_EDGE ( 'NONE', *, *, #14505, .F. ) ;
#29396=ORIENTED_EDGE ( 'NONE', *, *, #20446, .F. ) ;
#29407=CYLINDRICAL_SURFACE ( 'NONE', #26856, 20.00000000000001776 ) ;
#29424=CARTESIAN_POINT ( 'NONE',  ( 786.4999999999993179, 26.27639943461401018, 900.0000000000001137 ) ) ;
#29433=ORIENTED_EDGE ( 'NONE', *, *, #35997, .F. ) ;
#29494=VERTEX_POINT ( 'NONE', #15668 ) ;
#29514=CARTESIAN_POINT ( 'NONE',  ( -786.4999999999993179, -496.5085659523897448, -356.8883017825714319 ) ) ;
#29519=CARTESIAN_POINT ( 'NONE',  ( 746.4999999999993179, -365.3551492539851893, -8.132432514707076621 ) ) ;
#29528=LINE ( 'NONE', #43603, #4962 ) ;
#29557=EDGE_LOOP ( 'NONE', ( #15136, #33966 ) ) ;
#29629=LINE ( 'NONE', #9745, #27672 ) ;
#29632=DIRECTION ( 'NONE',  ( -1.000000000000000000, -0.000000000000000000, -0.000000000000000000 ) ) ;
#29646=VERTEX_POINT ( 'NONE', #36693 ) ;
#29667=DIRECTION ( 'NONE',  ( 0.000000000000000000, 0.000000000000000000, 1.000000000000000000 ) ) ;
#29676=DIRECTION ( 'NONE',  ( 0.000000000000000000, -0.9238795325112892920, 0.3826834323650836756 ) ) ;
#29678=CARTESIAN_POINT ( 'NONE',  ( -786.4999999999993179, -436.2161768796786987, 399.7184814855371542 ) ) ;
#29701=EDGE_LOOP ( 'NONE', ( #7882, #43608, #36363, #36250, #30970, #42624 ) ) ;
#29702=EDGE_CURVE ( 'NONE', #3542, #36764, #8477, .T. ) ;
#29708=VERTEX_POINT ( 'NONE', #2950 ) ;
#29720=FACE_OUTER_BOUND ( 'NONE', #14640, .T. ) ;
#29728=DIRECTION ( 'NONE',  ( 0.000000000000000000, 0.7372773368101331881, -0.6755902076156503622 ) ) ;
#29731=CARTESIAN_POINT ( 'NONE',  ( 775.4999999999993179, -501.1515549466498669, -368.0974687824633520 ) ) ;
#29744=VECTOR ( 'NONE', #35070, 1000.000000000000114 ) ;
#29773=EDGE_CURVE ( 'NONE', #44478, #30797, #14377, .T. ) ;
#29850=CARTESIAN_POINT ( 'NONE',  ( -37.63011601220122770, -513.1383975375929367, -349.9999999999999432 ) ) ;
#29854=LINE ( 'NONE', #19020, #11432 ) ;
#29862=EDGE_CURVE ( 'NONE', #36920, #12779, #3648, .T. ) ;
#29864=VECTOR ( 'NONE', #790, 1000.000000000000000 ) ;
#29882=EDGE_LOOP ( 'NONE', ( #44647, #26690, #4245, #4943 ) ) ;
#29893=DIRECTION ( 'NONE',  ( 1.000000000000000000, 0.000000000000000000, -0.000000000000000000 ) ) ;
#29906=DIRECTION ( 'NONE',  ( 1.000000000000000000, 0.000000000000000000, 0.000000000000000000 ) ) ;
#29914=DIRECTION ( 'NONE',  ( 0.000000000000000000, -0.3826834323650838976, -0.9238795325112892920 ) ) ;
#29946=EDGE_LOOP ( 'NONE', ( #31349, #16480, #43812, #27509 ) ) ;
#29951=AXIS2_PLACEMENT_3D ( 'NONE', #3837, #18167, #18612 ) ;
#29961=DIRECTION ( 'NONE',  ( 0.000000000000000000, 0.6755902076156502511, 0.7372773368101330771 ) ) ;
#29964=CARTESIAN_POINT ( 'NONE',  ( -746.4999999999993179, -365.3551492539851893, -28.13243251470704109 ) ) ;
#29986=LINE ( 'NONE', #19821, #19636 ) ;
#30000=EDGE_CURVE ( 'NONE', #36920, #2495, #28327, .T. ) ;
#30017=ORIENTED_EDGE ( 'NONE', *, *, #1266, .T. ) ;
#30056=EDGE_CURVE ( 'NONE', #17152, #34249, #35035, .T. ) ;
#30079=CARTESIAN_POINT ( 'NONE',  ( 784.4999999999993179, -501.1515549466498669, -368.0974687824633520 ) ) ;
#30084=DIRECTION ( 'NONE',  ( -0.000000000000000000, -0.6755902076156505842, -0.7372773368101327440 ) ) ;
#30089=EDGE_CURVE ( 'NONE', #757, #42387, #25096, .T. ) ;
#30097=CARTESIAN_POINT ( 'NONE',  ( -28.63011601220122415, -110.5936016518799221, 750.6326042729449455 ) ) ;
#30106=DIRECTION ( 'NONE',  ( 0.000000000000000000, 1.000000000000000000, 0.000000000000000000 ) ) ;
#30126=ORIENTED_EDGE ( 'NONE', *, *, #43588, .F. ) ;
#30193=EDGE_LOOP ( 'NONE', ( #6238, #749, #39855, #36647, #3776, #45699 ) ) ;
#30253=DIRECTION ( 'NONE',  ( 0.000000000000000000, 1.000000000000000000, 0.000000000000000000 ) ) ;
#30261=CARTESIAN_POINT ( 'NONE',  ( 773.4999999999993179, -365.3551492539851893, -18.13243251470705886 ) ) ;
#30278=VERTEX_POINT ( 'NONE', #29030 ) ;
#30305=ADVANCED_FACE ( 'NONE', ( #39896 ), #630, .F. ) ;
#30317=EDGE_CURVE ( 'NONE', #26139, #32281, #22307, .T. ) ;
#30323=CARTESIAN_POINT ( 'NONE',  ( -786.4999999999993179, -544.8427095258973623, -369.9999999999999432 ) ) ;
#30329=ORIENTED_EDGE ( 'NONE', *, *, #6342, .F. ) ;
#30332=EDGE_CURVE ( 'NONE', #29494, #34816, #21872, .T. ) ;
#30343=CARTESIAN_POINT ( 'NONE',  ( -39.63011601220123481, -513.1383975375929367, -349.9999999999999432 ) ) ;
#30355=DIRECTION ( 'NONE',  ( 0.000000000000000000, 0.000000000000000000, 1.000000000000000000 ) ) ;
#30358=PLANE ( 'NONE',  #26350 ) ;
#30376=CARTESIAN_POINT ( 'NONE',  ( 786.4999999999993179, 35.55895481007120651, 914.5706932916501728 ) ) ;
#30407=CARTESIAN_POINT ( 'NONE',  ( -775.4999999999993179, -496.5085659523897448, -356.8883017825714319 ) ) ;
#30412=CARTESIAN_POINT ( 'NONE',  ( -786.4999999999993179, -112.8054336623104348, 752.6593748957919843 ) ) ;
#30476=CIRCLE ( 'NONE', #6878, 10.00000000000000888 ) ;
#30488=VERTEX_POINT ( 'NONE', #30376 ) ;
#30495=CIRCLE ( 'NONE', #16494, 10.00000000000000888 ) ;
#30501=VERTEX_POINT ( 'NONE', #12156 ) ;
#30579=VECTOR ( 'NONE', #20266, 1000.000000000000114 ) ;
#30602=CLOSED_SHELL ( 'NONE', ( #38519, #40741, #1131, #42476, #45087, #38567, #22374, #13640, #35071, #34021, #43593, #30305, #22405, #19069, #43611, #2030, #3818, #20170, #19043, #18150, #9721, #32219, #36452, #39752 ) ) ;
#30606=EDGE_CURVE ( 'NONE', #44956, #38954, #36863, .T. ) ;
#30609=PLANE ( 'NONE',  #8480 ) ;
#30639=DIRECTION ( 'NONE',  ( 0.000000000000000000, 0.000000000000000000, 1.000000000000000000 ) ) ;
#30645=AXIS2_PLACEMENT_3D ( 'NONE', #31824, #35516, #3891 ) ;
#30646=AXIS2_PLACEMENT_3D ( 'NONE', #33645, #1998, #30639 ) ;
#30648=DIRECTION ( 'NONE',  ( 1.000000000000000000, 0.000000000000000000, 0.000000000000000000 ) ) ;
#30650=DIRECTION ( 'NONE',  ( -1.000000000000000000, 0.000000000000000000, 0.000000000000000000 ) ) ;
#30657=DIRECTION ( 'NONE',  ( 1.000000000000000000, 0.000000000000000000, 0.000000000000000000 ) ) ;
#30700=VERTEX_POINT ( 'NONE', #24127 ) ;
#30715=DIRECTION ( 'NONE',  ( -1.000000000000000000, -0.000000000000000000, 0.000000000000000000 ) ) ;
#30721=DIRECTION ( 'NONE',  ( -0.000000000000000000, 0.3826834323650978309, 0.9238795325112835188 ) ) ;
#30735=CARTESIAN_POINT ( 'NONE',  ( -26.63011601220122060, -512.9681489794448908, -339.9999999999999432 ) ) ;
#30751=ORIENTED_EDGE ( 'NONE', *, *, #24955, .F. ) ;
#30756=ORIENTED_EDGE ( 'NONE', *, *, #45316, .F. ) ;
#30758=VECTOR ( 'NONE', #17120, 1000.000000000000114 ) ;
#30787=AXIS2_PLACEMENT_3D ( 'NONE', #36358, #18821, #18593 ) ;
#30797=VERTEX_POINT ( 'NONE', #17203 ) ;
#30803=VERTEX_POINT ( 'NONE', #7048 ) ;
#30810=DIRECTION ( 'NONE',  ( 1.000000000000000000, -0.000000000000000000, -0.000000000000000000 ) ) ;
#30814=DIRECTION ( 'NONE',  ( 1.000000000000000000, 0.000000000000000000, -0.000000000000000000 ) ) ;
#30837=CARTESIAN_POINT ( 'NONE',  ( -26.63011601220122060, -544.8427095258973623, -350.0000000000000000 ) ) ;
#30845=ORIENTED_EDGE ( 'NONE', *, *, #7440, .F. ) ;
#30851=FACE_OUTER_BOUND ( 'NONE', #9780, .T. ) ;
#30867=CARTESIAN_POINT ( 'NONE',  ( 784.4999999999993179, -501.1515549466498669, -368.0974687824633520 ) ) ;
#30893=EDGE_LOOP ( 'NONE', ( #39331, #30751, #42330, #25216 ) ) ;
#30914=ORIENTED_EDGE ( 'NONE', *, *, #9097, .F. ) ;
#30970=ORIENTED_EDGE ( 'NONE', *, *, #30056, .F. ) ;
#31012=ORIENTED_EDGE ( 'NONE', *, *, #25157, .T. ) ;
#31017=ORIENTED_EDGE ( 'NONE', *, *, #4891, .T. ) ;
#31022=VERTEX_POINT ( 'NONE', #22040 ) ;
#31034=DIRECTION ( 'NONE',  ( 0.000000000000000000, 0.000000000000000000, 1.000000000000000000 ) ) ;
#31038=LINE ( 'NONE', #34511, #34938 ) ;
#31108=MECHANICAL_DESIGN_GEOMETRIC_PRESENTATION_REPRESENTATION('',(#19308),#32608);
#31116=DIRECTION ( 'NONE',  ( -1.000000000000000000, -0.000000000000000000, -0.000000000000000000 ) ) ;
#31204=CARTESIAN_POINT ( 'NONE',  ( -39.63011601220123481, -494.6608068873671300, -357.6536686473015720 ) ) ;
#31216=EDGE_CURVE ( 'NONE', #26139, #34942, #34344, .T. ) ;
#31245=DIRECTION ( 'NONE',  ( 0.000000000000000000, 0.9238795325112891810, -0.3826834323650838421 ) ) ;
#31246=VERTEX_POINT ( 'NONE', #42615 ) ;
#31248=CIRCLE ( 'NONE', #23382, 9.999999999999982236 ) ;
#31249=ORIENTED_EDGE ( 'NONE', *, *, #25229, .T. ) ;
#31289=CARTESIAN_POINT ( 'NONE',  ( -746.4999999999993179, -365.3551492539851893, -8.132432514707076621 ) ) ;
#31297=CARTESIAN_POINT ( 'NONE',  ( -746.4999999999993179, -365.3551492539851893, -18.13243251470705886 ) ) ;
#31323=DIRECTION ( 'NONE',  ( -1.000000000000000000, -0.000000000000000000, -0.000000000000000000 ) ) ;
#31349=ORIENTED_EDGE ( 'NONE', *, *, #19921, .F. ) ;
#31403=DIRECTION ( 'NONE',  ( 1.000000000000000000, 0.000000000000000000, -0.000000000000000000 ) ) ;
#31448=VECTOR ( 'NONE', #23973, 1000.000000000000000 ) ;
#31452=CARTESIAN_POINT ( 'NONE',  ( 775.4999999999993179, -110.5936016518799221, 750.6326042729449455 ) ) ;
#31495=CARTESIAN_POINT ( 'NONE',  ( 784.4999999999993179, -496.5085659523897448, -356.8883017825714319 ) ) ;
#31524=CARTESIAN_POINT ( 'NONE',  ( -26.63011601220122060, -512.9681489794448908, -329.9999999999999432 ) ) ;
#31530=EDGE_CURVE ( 'NONE', #16954, #3483, #9075, .T. ) ;
#31539=DIRECTION ( 'NONE',  ( -1.000000000000000000, -0.000000000000000000, -0.000000000000000000 ) ) ;
#31549=ORIENTED_EDGE ( 'NONE', *, *, #33987, .T. ) ;
#31569=DIRECTION ( 'NONE',  ( 0.000000000000000000, 0.000000000000000000, 1.000000000000000000 ) ) ;
#31579=EDGE_LOOP ( 'NONE', ( #6138, #6503, #41146, #40953 ) ) ;
#31585=DIRECTION ( 'NONE',  ( 0.000000000000000000, 0.000000000000000000, 1.000000000000000000 ) ) ;
#31609=AXIS2_PLACEMENT_3D ( 'NONE', #33176, #8697, #37700 ) ;
#31644=EDGE_LOOP ( 'NONE', ( #14694, #18823, #44062, #33631 ) ) ;
#31655=LINE ( 'NONE', #3497, #32920 ) ;
#31660=EDGE_LOOP ( 'NONE', ( #13925, #18996 ) ) ;
#31662=FACE_OUTER_BOUND ( 'NONE', #24888, .T. ) ;
#31689=ORIENTED_EDGE ( 'NONE', *, *, #37580, .F. ) ;
#31709=DIRECTION ( 'NONE',  ( 0.000000000000000000, 0.000000000000000000, 1.000000000000000000 ) ) ;
#31713=DIRECTION ( 'NONE',  ( 0.000000000000000000, 0.000000000000000000, 1.000000000000000000 ) ) ;
#31774=DIRECTION ( 'NONE',  ( -1.000000000000000000, -0.000000000000000000, -0.000000000000000000 ) ) ;
#31782=EDGE_CURVE ( 'NONE', #40120, #4703, #22925, .T. ) ;
#31786=CARTESIAN_POINT ( 'NONE',  ( 784.4999999999993179, -365.3551492539851893, -18.13243251470705886 ) ) ;
#31793=CARTESIAN_POINT ( 'NONE',  ( -26.63011601220122060, -512.9681489794448908, -339.9999999999999432 ) ) ;
#31803=DIRECTION ( 'NONE',  ( 0.000000000000000000, 0.000000000000000000, -1.000000000000000000 ) ) ;
#31806=ORIENTED_EDGE ( 'NONE', *, *, #39951, .F. ) ;
#31824=CARTESIAN_POINT ( 'NONE',  ( 773.4999999999993179, -365.3551492539851893, -18.13243251470705886 ) ) ;
#31830=DIRECTION ( 'NONE',  ( 0.000000000000000000, 0.3826834323650836756, 0.9238795325112892920 ) ) ;
#31880=ORIENTED_EDGE ( 'NONE', *, *, #169, .T. ) ;
#31892=AXIS2_PLACEMENT_3D ( 'NONE', #45611, #7024, #21113 ) ;
#31918=ORIENTED_EDGE ( 'NONE', *, *, #24423, .F. ) ;
#31941=DIRECTION ( 'NONE',  ( 0.000000000000000000, -0.3826834323650835645, -0.9238795325112892920 ) ) ;
#31963=CARTESIAN_POINT ( 'NONE',  ( -26.63011601220122060, -110.5936016518799221, 750.6326042729449455 ) ) ;
#31973=PLANE ( 'NONE',  #30787 ) ;
#31992=CARTESIAN_POINT ( 'NONE',  ( -773.4999999999993179, -512.9681489794448908, -350.0000000000000000 ) ) ;
#32002=DIRECTION ( 'NONE',  ( -0.000000000000000000, -0.000000000000000000, -1.000000000000000000 ) ) ;
#32007=DIRECTION ( 'NONE',  ( -1.000000000000000000, -0.000000000000000000, 0.000000000000000000 ) ) ;
#32011=EDGE_CURVE ( 'NONE', #40960, #12731, #4136, .T. ) ;
#32013=DIRECTION ( 'NONE',  ( 0.000000000000000000, 0.000000000000000000, 1.000000000000000000 ) ) ;
#32020=DIRECTION ( 'NONE',  ( 0.000000000000000000, 0.000000000000000000, 1.000000000000000000 ) ) ;
#32082=DIRECTION ( 'NONE',  ( 1.000000000000000000, 0.000000000000000000, 0.000000000000000000 ) ) ;
#32093=AXIS2_PLACEMENT_3D ( 'NONE', #17825, #10659, #18054 ) ;
#32094=EDGE_CURVE ( 'NONE', #12779, #7478, #14146, .T. ) ;
#32125=AXIS2_PLACEMENT_3D ( 'NONE', #15215, #7364, #43377 ) ;
#32176=ORIENTED_EDGE ( 'NONE', *, *, #18259, .T. ) ;
#32191=LINE ( 'NONE', #22020, #21685 ) ;
#32193=FACE_BOUND ( 'NONE', #6538, .T. ) ;
#32195=DIRECTION ( 'NONE',  ( 1.000000000000000000, -0.000000000000000000, -0.000000000000000000 ) ) ;
#32207=CIRCLE ( 'NONE', #13789, 9.999999999999982236 ) ;
#32219=ADVANCED_FACE ( 'NONE', ( #19148 ), #11546, .T. ) ;
#32223=ORIENTED_EDGE ( 'NONE', *, *, #24269, .T. ) ;
#32243=LINE ( 'NONE', #14704, #24774 ) ;
#32248=FACE_OUTER_BOUND ( 'NONE', #2381, .T. ) ;
#32264=EDGE_CURVE ( 'NONE', #25758, #42149, #18932, .T. ) ;
#32270=VECTOR ( 'NONE', #43162, 1000.000000000000000 ) ;
#32281=VERTEX_POINT ( 'NONE', #5056 ) ;
#32316=VECTOR ( 'NONE', #8360, 1000.000000000000000 ) ;
#32324=CYLINDRICAL_SURFACE ( 'NONE', #1132, 12.00000000000001066 ) ;
#32328=DIRECTION ( 'NONE',  ( 0.000000000000000000, 0.000000000000000000, 1.000000000000000000 ) ) ;
#32355=VERTEX_POINT ( 'NONE', #40166 ) ;
#32375=EDGE_CURVE ( 'NONE', #7404, #69, #29986, .T. ) ;
#32379=CARTESIAN_POINT ( 'NONE',  ( -786.4999999999993179, 26.27639943461401018, 900.0000000000001137 ) ) ;
#32381=AXIS2_PLACEMENT_3D ( 'NONE', #3860, #17950, #32020 ) ;
#32405=DIRECTION ( 'NONE',  ( -0.000000000000000000, 0.000000000000000000, 1.000000000000000000 ) ) ;
#32451=VERTEX_POINT ( 'NONE', #19587 ) ;
#32461=ORIENTED_EDGE ( 'NONE', *, *, #6908, .F. ) ;
#32482=DIRECTION ( 'NONE',  ( 0.000000000000000000, 0.3826834323650838421, 0.9238795325112891810 ) ) ;
#32491=DIRECTION ( 'NONE',  ( 0.000000000000000000, 0.3826834323650836200, 0.9238795325112892920 ) ) ;
#32557=DIRECTION ( 'NONE',  ( 0.000000000000000000, -0.3826834323650836756, -0.9238795325112892920 ) ) ;
#32566=ORIENTED_EDGE ( 'NONE', *, *, #31216, .T. ) ;
#32583=ADVANCED_FACE ( 'NONE', ( #40407 ), #44775, .F. ) ;
#32603=DIRECTION ( 'NONE',  ( 1.000000000000000000, 0.000000000000000000, 0.000000000000000000 ) ) ;
#32608=( GEOMETRIC_REPRESENTATION_CONTEXT ( 3 ) GLOBAL_UNCERTAINTY_ASSIGNED_CONTEXT ( ( #37024 ) ) GLOBAL_UNIT_ASSIGNED_CONTEXT ( ( #32820, #15041, #35826 ) ) REPRESENTATION_CONTEXT ( 'NONE', 'WORKASPACE' ) );
#32627=EDGE_CURVE ( 'NONE', #35816, #22668, #9433, .T. ) ;
#32650=FACE_OUTER_BOUND ( 'NONE', #5915, .T. ) ;
#32693=PLANE ( 'NONE',  #16654 ) ;
#32703=CARTESIAN_POINT ( 'NONE',  ( -784.4999999999993179, -513.1383975375929367, -369.9999999999999432 ) ) ;
#32726=EDGE_LOOP ( 'NONE', ( #9103, #13190, #8099, #5622 ) ) ;
#32754=FACE_OUTER_BOUND ( 'NONE', #35190, .T. ) ;
#32764=ORIENTED_EDGE ( 'NONE', *, *, #37597, .T. ) ;
#32765=VECTOR ( 'NONE', #38675, 1000.000000000000000 ) ;
#32812=VERTEX_POINT ( 'NONE', #42209 ) ;
#32820=( LENGTH_UNIT ( ) NAMED_UNIT ( * ) SI_UNIT ( .MILLI., .METRE. ) );
#32825=CARTESIAN_POINT ( 'NONE',  ( -775.4999999999993179, -563.3203001761230553, -342.3463313526983143 ) ) ;
#32862=EDGE_CURVE ( 'NONE', #29646, #40310, #30476, .T. ) ;
#32865=AXIS2_PLACEMENT_3D ( 'NONE', #23990, #30721, #45502 ) ;
#32869=CARTESIAN_POINT ( 'NONE',  ( -28.63011601220122415, -365.3551492539851893, -8.132432514707076621 ) ) ;
#32872=EDGE_CURVE ( 'NONE', #18154, #32812, #36393, .T. ) ;
#32873=ORIENTED_EDGE ( 'NONE', *, *, #20771, .F. ) ;
#32879=DIRECTION ( 'NONE',  ( -1.000000000000000000, -0.000000000000000000, -0.000000000000000000 ) ) ;
#32881=AXIS2_PLACEMENT_3D ( 'NONE', #31963, #14895, #39618 ) ;
#32894=ADVANCED_FACE ( 'NONE', ( #34813 ), #3870, .F. ) ;
#32897=VECTOR ( 'NONE', #35407, 999.9999999999998863 ) ;
#32920=VECTOR ( 'NONE', #20404, 1000.000000000000000 ) ;
#32924=EDGE_LOOP ( 'NONE', ( #14956, #35277 ) ) ;
#32943=DIRECTION ( 'NONE',  ( 0.000000000000000000, 0.000000000000000000, 1.000000000000000000 ) ) ;
#32957=EDGE_CURVE ( 'NONE', #45720, #4703, #15752, .T. ) ;
#32996=DIRECTION ( 'NONE',  ( 1.000000000000000000, -0.000000000000000000, -0.000000000000000000 ) ) ;
#33002=DIRECTION ( 'NONE',  ( 0.000000000000000000, 0.3826834323650836756, 0.9238795325112892920 ) ) ;
#33015=EDGE_LOOP ( 'NONE', ( #22107, #6481, #10563, #25830 ) ) ;
#33050=DIRECTION ( 'NONE',  ( 1.000000000000000000, -0.000000000000000000, -0.000000000000000000 ) ) ;
#33065=DIRECTION ( 'NONE',  ( 1.000000000000000000, 0.000000000000000000, -0.000000000000000000 ) ) ;
#33102=CARTESIAN_POINT ( 'NONE',  ( -779.9999999999993179, -513.1383975375929367, -367.9999999999999432 ) ) ;
#33106=VECTOR ( 'NONE', #27759, 1000.000000000000000 ) ;
#33107=CARTESIAN_POINT ( 'NONE',  ( 786.4999999999993179, -365.3551492539851893, -18.13243251470705886 ) ) ;
#33115=CARTESIAN_POINT ( 'NONE',  ( -784.4999999999993179, 22.32581219114657856, 895.6886905569881492 ) ) ;
#33153=LINE ( 'NONE', #12125, #22592 ) ;
#33176=CARTESIAN_POINT ( 'NONE',  ( -773.4999999999993179, -512.9681489794448908, -339.9999999999999432 ) ) ;
#33191=ORIENTED_EDGE ( 'NONE', *, *, #16139, .T. ) ;
#33200=EDGE_CURVE ( 'NONE', #16297, #14962, #40785, .T. ) ;
#33206=EDGE_CURVE ( 'NONE', #42149, #19960, #23667, .T. ) ;
#33250=ORIENTED_EDGE ( 'NONE', *, *, #4320, .F. ) ;
#33261=VERTEX_POINT ( 'NONE', #44019 ) ;
#33295=VERTEX_POINT ( 'NONE', #44252 ) ;
#33319=CARTESIAN_POINT ( 'NONE',  ( 786.4999999999993179, -544.8427095258973623, -350.0000000000000000 ) ) ;
#33326=LINE ( 'NONE', #29424, #26888 ) ;
#33327=LINE ( 'NONE', #44872, #8493 ) ;
#33340=DIRECTION ( 'NONE',  ( 1.000000000000000000, -0.000000000000000000, -0.000000000000000000 ) ) ;
#33348=ORIENTED_EDGE ( 'NONE', *, *, #33200, .T. ) ;
#33382=CIRCLE ( 'NONE', #31892, 9.999999999999982236 ) ;
#33391=MANIFOLD_SOLID_BREP ( 'Boss-Extrude22', #7004 ) ;
#33421=EDGE_CURVE ( 'NONE', #22668, #518, #41710, .T. ) ;
#33427=ORIENTED_EDGE ( 'NONE', *, *, #9097, .T. ) ;
#33444=ORIENTED_EDGE ( 'NONE', *, *, #13291, .F. ) ;
#33451=ORIENTED_EDGE ( 'NONE', *, *, #2313, .F. ) ;
#33465=AXIS2_PLACEMENT_3D ( 'NONE', #40089, #33837, #1959 ) ;
#33493=CARTESIAN_POINT ( 'NONE',  ( -37.63011601220122770, -544.8427095258973623, -369.9999999999999432 ) ) ;
#33510=ADVANCED_FACE ( 'NONE', ( #30851 ), #20891, .T. ) ;
#33518=CIRCLE ( 'NONE', #44569, 9.999999999999982236 ) ;
#33533=CARTESIAN_POINT ( 'NONE',  ( -66.63011601220125613, -365.3551492539851893, -18.13243251470705886 ) ) ;
#33540=LINE ( 'NONE', #30079, #7685 ) ;
#33542=CARTESIAN_POINT ( 'NONE',  ( 784.4999999999993179, -563.3203001761230553, -342.3463313526983143 ) ) ;
#33573=ORIENTED_EDGE ( 'NONE', *, *, #19601, .T. ) ;
#33578=CIRCLE ( 'NONE', #13676, 9.999999999999982236 ) ;
#33585=LINE ( 'NONE', #19266, #37316 ) ;
#33597=FACE_OUTER_BOUND ( 'NONE', #25584, .T. ) ;
#33629=( NAMED_UNIT ( * ) SI_UNIT ( $, .STERADIAN. ) SOLID_ANGLE_UNIT ( ) );
#33631=ORIENTED_EDGE ( 'NONE', *, *, #16139, .F. ) ;
#33638=CIRCLE ( 'NONE', #41769, 20.00000000000001776 ) ;
#33639=ORIENTED_EDGE ( 'NONE', *, *, #11876, .T. ) ;
#33645=CARTESIAN_POINT ( 'NONE',  ( 784.4999999999993179, -544.8427095258973623, -350.0000000000000000 ) ) ;
#33660=EDGE_CURVE ( 'NONE', #45642, #41202, #31248, .T. ) ;
#33663=ORIENTED_EDGE ( 'NONE', *, *, #37065, .F. ) ;
#33679=ORIENTED_EDGE ( 'NONE', *, *, #20069, .F. ) ;
#33705=ORIENTED_EDGE ( 'NONE', *, *, #20446, .T. ) ;
#33711=CARTESIAN_POINT ( 'NONE',  ( -37.63011601220122770, -365.3551492539851893, -28.13243251470704109 ) ) ;
#33715=VERTEX_POINT ( 'NONE', #45169 ) ;
#33738=ADVANCED_FACE ( 'NONE', ( #3121 ), #17210, .F. ) ;
#33740=DIRECTION ( 'NONE',  ( -1.000000000000000000, -0.000000000000000000, 0.000000000000000000 ) ) ;
#33744=VECTOR ( 'NONE', #35472, 1000.000000000000000 ) ;
#33752=AXIS2_PLACEMENT_3D ( 'NONE', #8597, #19423, #22663 ) ;
#33753=ORIENTED_EDGE ( 'NONE', *, *, #4642, .F. ) ;
#33761=ADVANCED_FACE ( 'NONE', ( #25275 ), #36139, .T. ) ;
#33816=LINE ( 'NONE', #26431, #6349 ) ;
#33831=DIRECTION ( 'NONE',  ( 0.000000000000000000, -0.3826834323650837866, -0.9238795325112891810 ) ) ;
#33837=DIRECTION ( 'NONE',  ( 0.000000000000000000, -0.9238795325112892920, 0.3826834323650836756 ) ) ;
#33856=DIRECTION ( 'NONE',  ( -0.000000000000000000, -0.000000000000000000, -1.000000000000000000 ) ) ;
#33879=CARTESIAN_POINT ( 'NONE',  ( -26.63011601220122060, -513.1383975375929367, -369.9999999999999432 ) ) ;
#33966=ORIENTED_EDGE ( 'NONE', *, *, #2367, .F. ) ;
#33979=ORIENTED_EDGE ( 'NONE', *, *, #13335, .F. ) ;
#33987=EDGE_CURVE ( 'NONE', #22437, #2273, #21961, .T. ) ;
#34021=ADVANCED_FACE ( 'NONE', ( #22048, #11663, #25739 ), #31973, .F. ) ;
#34031=DIRECTION ( 'NONE',  ( 0.000000000000000000, 0.000000000000000000, 1.000000000000000000 ) ) ;
#34053=CARTESIAN_POINT ( 'NONE',  ( 1007.605605532488426, 35.55895481007120651, 914.5706932916501728 ) ) ;
#34054=LINE ( 'NONE', #9121, #43778 ) ;
#34068=ORIENTED_EDGE ( 'NONE', *, *, #4642, .T. ) ;
#34071=AXIS2_PLACEMENT_3D ( 'NONE', #611, #22515, #29013 ) ;
#34107=DIRECTION ( 'NONE',  ( 0.000000000000000000, 0.9238795325112891810, -0.3826834323650838421 ) ) ;
#34144=ORIENTED_EDGE ( 'NONE', *, *, #2947, .F. ) ;
#34160=VECTOR ( 'NONE', #33856, 1000.000000000000000 ) ;
#34185=ORIENTED_EDGE ( 'NONE', *, *, #23904, .T. ) ;
#34210=( GEOMETRIC_REPRESENTATION_CONTEXT ( 3 ) GLOBAL_UNCERTAINTY_ASSIGNED_CONTEXT ( ( #36592 ) ) GLOBAL_UNIT_ASSIGNED_CONTEXT ( ( #43968, #37497, #1925 ) ) REPRESENTATION_CONTEXT ( 'NONE', 'WORKASPACE' ) );
#34215=DIRECTION ( 'NONE',  ( 1.000000000000000000, 0.000000000000000000, 0.000000000000000000 ) ) ;
#34236=DIRECTION ( 'NONE',  ( 0.000000000000000000, 0.3826834323650836756, 0.9238795325112892920 ) ) ;
#34239=ADVANCED_FACE ( 'NONE', ( #22484 ), #43963, .F. ) ;
#34241=DIRECTION ( 'NONE',  ( 0.000000000000000000, 0.000000000000000000, 1.000000000000000000 ) ) ;
#34249=VERTEX_POINT ( 'NONE', #30323 ) ;
#34252=VECTOR ( 'NONE', #32195, 1000.000000000000000 ) ;
#34271=CARTESIAN_POINT ( 'NONE',  ( -26.63011601220122060, -110.5936016518799221, 750.6326042729449455 ) ) ;
#34275=DIRECTION ( 'NONE',  ( 0.000000000000000000, 0.000000000000000000, -1.000000000000000000 ) ) ;
#34279=DIRECTION ( 'NONE',  ( 0.000000000000000000, 0.000000000000000000, 1.000000000000000000 ) ) ;
#34287=DIRECTION ( 'NONE',  ( 1.000000000000000000, -0.000000000000000000, -0.000000000000000000 ) ) ;
#34294=CARTESIAN_POINT ( 'NONE',  ( 786.4999999999993179, 26.27639943461418426, 900.0000000000004547 ) ) ;
#34298=VERTEX_POINT ( 'NONE', #5168 ) ;
#34328=AXIS2_PLACEMENT_3D ( 'NONE', #30735, #16180, #20096 ) ;
#34337=CARTESIAN_POINT ( 'NONE',  ( -775.4999999999993179, -513.1383975375929367, -369.9999999999999432 ) ) ;
#34340=ORIENTED_EDGE ( 'NONE', *, *, #1266, .F. ) ;
#34344=CIRCLE ( 'NONE', #24745, 20.00000000000001776 ) ;
#34348=DIRECTION ( 'NONE',  ( 1.000000000000000000, 0.000000000000000000, -0.000000000000000000 ) ) ;
#34357=DIRECTION ( 'NONE',  ( 1.000000000000000000, 0.000000000000000000, 0.000000000000000000 ) ) ;
#34371=ORIENTED_EDGE ( 'NONE', *, *, #13291, .T. ) ;
#34374=AXIS2_PLACEMENT_3D ( 'NONE', #8969, #40618, #13133 ) ;
#34395=VECTOR ( 'NONE', #35873, 999.9999999999998863 ) ;
#34451=VERTEX_POINT ( 'NONE', #8654 ) ;
#34468=AXIS2_PLACEMENT_3D ( 'NONE', #17489, #38972, #34572 ) ;
#34511=CARTESIAN_POINT ( 'NONE',  ( -786.4999999999993179, -544.8427095258973623, -369.9999999999999432 ) ) ;
#34534=DIRECTION ( 'NONE',  ( 0.000000000000000000, 1.000000000000000000, 0.000000000000000000 ) ) ;
#34559=DIRECTION ( 'NONE',  ( 0.000000000000000000, 0.000000000000000000, 1.000000000000000000 ) ) ;
#34560=DIRECTION ( 'NONE',  ( -1.000000000000000000, -0.000000000000000000, -0.000000000000000000 ) ) ;
#34572=DIRECTION ( 'NONE',  ( -1.000000000000000000, 0.000000000000000000, 0.000000000000000000 ) ) ;
#34583=DIRECTION ( 'NONE',  ( 0.000000000000000000, 0.000000000000000000, 1.000000000000000000 ) ) ;
#34601=ADVANCED_FACE ( 'NONE', ( #35166 ), #3545, .F. ) ;
#34612=EDGE_CURVE ( 'NONE', #30278, #22547, #41882, .T. ) ;
#34623=DIRECTION ( 'NONE',  ( 1.000000000000000000, 0.000000000000000000, -0.000000000000000000 ) ) ;
#34626=CARTESIAN_POINT ( 'NONE',  ( -784.4999999999993179, -365.3551492539851893, -28.13243251470704109 ) ) ;
#34639=DIRECTION ( 'NONE',  ( 1.000000000000000000, 0.000000000000000000, -0.000000000000000000 ) ) ;
#34654=ADVANCED_FACE ( 'NONE', ( #10451 ), #16711, .F. ) ;
#34680=DIRECTION ( 'NONE',  ( -0.000000000000000000, 0.000000000000000000, 1.000000000000000000 ) ) ;
#34688=DIRECTION ( 'NONE',  ( -1.000000000000000000, -0.000000000000000000, 0.000000000000000000 ) ) ;
#34704=ORIENTED_EDGE ( 'NONE', *, *, #9784, .F. ) ;
#34713=ORIENTED_EDGE ( 'NONE', *, *, #2708, .F. ) ;
#34716=ORIENTED_EDGE ( 'NONE', *, *, #43588, .T. ) ;
#34722=CARTESIAN_POINT ( 'NONE',  ( -786.4999999999993179, -544.8427095258973623, -350.0000000000000000 ) ) ;
#34723=LINE ( 'NONE', #41212, #36851 ) ;
#34727=FACE_OUTER_BOUND ( 'NONE', #16034, .T. ) ;
#34741=DIRECTION ( 'NONE',  ( 1.000000000000000000, 0.000000000000000000, -0.000000000000000000 ) ) ;
#34761=VERTEX_POINT ( 'NONE', #13474 ) ;
#34808=AXIS2_PLACEMENT_3D ( 'NONE', #27884, #2472, #38498 ) ;
#34813=FACE_OUTER_BOUND ( 'NONE', #22806, .T. ) ;
#34816=VERTEX_POINT ( 'NONE', #24304 ) ;
#34903=CARTESIAN_POINT ( 'NONE',  ( -66.63011601220125613, -365.3551492539851893, -8.132432514707076621 ) ) ;
#34912=DIRECTION ( 'NONE',  ( -1.000000000000000000, -0.000000000000000000, -0.000000000000000000 ) ) ;
#34938=VECTOR ( 'NONE', #24328, 1000.000000000000000 ) ;
#34942=VERTEX_POINT ( 'NONE', #526 ) ;
#34952=CARTESIAN_POINT ( 'NONE',  ( -786.4999999999993179, 323.4107432173689176, 352.9408934102648345 ) ) ;
#34969=DIRECTION ( 'NONE',  ( 1.000000000000000000, -0.000000000000000000, -0.000000000000000000 ) ) ;
#34975=DIRECTION ( 'NONE',  ( 0.000000000000000000, 0.000000000000000000, 1.000000000000000000 ) ) ;
#35004=DIRECTION ( 'NONE',  ( 0.000000000000000000, 0.3826834323650836756, 0.9238795325112892920 ) ) ;
#35019=CYLINDRICAL_SURFACE ( 'NONE', #35609, 10.00000000000000888 ) ;
#35031=VERTEX_POINT ( 'NONE', #39800 ) ;
#35035=CIRCLE ( 'NONE', #16587, 19.99999999999990763 ) ;
#35070=DIRECTION ( 'NONE',  ( -0.000000000000000000, -0.6755902076156505842, -0.7372773368101328550 ) ) ;
#35071=ADVANCED_FACE ( 'NONE', ( #42321 ), #28704, .F. ) ;
#35089=CARTESIAN_POINT ( 'NONE',  ( -746.4999999999993179, -355.4967352946684969, -16.45562775363632113 ) ) ;
#35102=CIRCLE ( 'NONE', #18909, 19.99999999999990763 ) ;
#35166=FACE_OUTER_BOUND ( 'NONE', #25568, .T. ) ;
#35168=ORIENTED_EDGE ( 'NONE', *, *, #22408, .T. ) ;
#35171=EDGE_CURVE ( 'NONE', #10285, #39064, #7229, .T. ) ;
#35174=AXIS2_PLACEMENT_3D ( 'NONE', #24901, #10588, #35518 ) ;
#35186=EDGE_LOOP ( 'NONE', ( #33663, #33979 ) ) ;
#35190=EDGE_LOOP ( 'NONE', ( #22352, #7122, #19909, #14275 ) ) ;
#35232=ORIENTED_EDGE ( 'NONE', *, *, #28077, .F. ) ;
#35262=CYLINDRICAL_SURFACE ( 'NONE', #15266, 9.999999999999980460 ) ;
#35267=AXIS2_PLACEMENT_3D ( 'NONE', #45680, #44761, #20495 ) ;
#35277=ORIENTED_EDGE ( 'NONE', *, *, #15930, .F. ) ;
#35296=CIRCLE ( 'NONE', #21287, 12.00000000000001066 ) ;
#35299=CARTESIAN_POINT ( 'NONE',  ( -786.4999999999993179, -110.5936016518799221, 750.6326042729449455 ) ) ;
#35330=EDGE_CURVE ( 'NONE', #1374, #40310, #43682, .T. ) ;
#35382=ADVANCED_FACE ( 'NONE', ( #26125 ), #40240, .T. ) ;
#35395=ORIENTED_EDGE ( 'NONE', *, *, #32872, .F. ) ;
#35405=ORIENTED_EDGE ( 'NONE', *, *, #17918, .F. ) ;
#35407=DIRECTION ( 'NONE',  ( 0.000000000000000000, 0.7372773368101421809, -0.6755902076156404812 ) ) ;
#35409=EDGE_CURVE ( 'NONE', #4454, #22319, #26575, .T. ) ;
#35429=EDGE_CURVE ( 'NONE', #11840, #3483, #3021, .T. ) ;
#35434=PLANE ( 'NONE',  #32881 ) ;
#35472=DIRECTION ( 'NONE',  ( 0.000000000000000000, 1.000000000000000000, 0.000000000000000000 ) ) ;
#35473=CARTESIAN_POINT ( 'NONE',  ( -26.63011601220122060, -512.9681489794448908, -339.9999999999999432 ) ) ;
#35477=DIRECTION ( 'NONE',  ( 1.000000000000000000, -0.000000000000000000, -0.000000000000000000 ) ) ;
#35478=CARTESIAN_POINT ( 'NONE',  ( 786.4999999999993179, -295.7697417039441916, 122.5118383533586837 ) ) ;
#35486=FACE_OUTER_BOUND ( 'NONE', #2391, .T. ) ;
#35516=DIRECTION ( 'NONE',  ( -1.000000000000000000, -0.000000000000000000, 0.000000000000000000 ) ) ;
#35518=DIRECTION ( 'NONE',  ( 0.000000000000000000, 0.000000000000000000, -1.000000000000000000 ) ) ;
#35553=CIRCLE ( 'NONE', #17134, 10.00000000000000888 ) ;
#35554=CARTESIAN_POINT ( 'NONE',  ( 786.4999999999993179, -494.6608068873671300, -357.6536686473015720 ) ) ;
#35564=EDGE_LOOP ( 'NONE', ( #10176, #13725, #45002, #12828 ) ) ;
#35579=CARTESIAN_POINT ( 'NONE',  ( 786.4999999999993179, -494.6608068873671300, -357.6536686473015720 ) ) ;
#35589=LINE ( 'NONE', #3965, #33106 ) ;
#35609=AXIS2_PLACEMENT_3D ( 'NONE', #35473, #3152, #27876 ) ;
#35634=ORIENTED_EDGE ( 'NONE', *, *, #25229, .F. ) ;
#35695=VECTOR ( 'NONE', #31941, 1000.000000000000114 ) ;
#35714=LINE ( 'NONE', #14031, #41269 ) ;
#35742=EDGE_CURVE ( 'NONE', #19577, #2495, #11, .T. ) ;
#35749=AXIS2_PLACEMENT_3D ( 'NONE', #16454, #26400, #6053 ) ;
#35781=DIRECTION ( 'NONE',  ( -1.000000000000000000, -0.000000000000000000, 0.000000000000000000 ) ) ;
#35813=CARTESIAN_POINT ( 'NONE',  ( -66.63011601220125613, -365.3551492539851893, -28.13243251470704109 ) ) ;
#35816=VERTEX_POINT ( 'NONE', #28649 ) ;
#35826=( NAMED_UNIT ( * ) SI_UNIT ( $, .STERADIAN. ) SOLID_ANGLE_UNIT ( ) );
#35836=DIRECTION ( 'NONE',  ( 0.000000000000000000, -0.9238795325112835188, 0.3826834323650978309 ) ) ;
#35857=ORIENTED_EDGE ( 'NONE', *, *, #17371, .T. ) ;
#35873=DIRECTION ( 'NONE',  ( 0.000000000000000000, -0.9238795325112835188, 0.3826834323650978309 ) ) ;
#35884=FACE_OUTER_BOUND ( 'NONE', #41421, .T. ) ;
#35897=ORIENTED_EDGE ( 'NONE', *, *, #9784, .T. ) ;
#35899=VECTOR ( 'NONE', #4577, 1000.000000000000000 ) ;
#35927=DIRECTION ( 'NONE',  ( 0.000000000000000000, -0.3826834323650838421, -0.9238795325112891810 ) ) ;
#35932=DIRECTION ( 'NONE',  ( -1.000000000000000000, -0.000000000000000000, -0.000000000000000000 ) ) ;
#35937=DIRECTION ( 'NONE',  ( 0.000000000000000000, 0.000000000000000000, -1.000000000000000000 ) ) ;
#35989=CARTESIAN_POINT ( 'NONE',  ( -66.63011601220125613, -365.3551492539851893, -18.13243251470705886 ) ) ;
#35997=EDGE_CURVE ( 'NONE', #601, #42149, #11318, .T. ) ;
#36000=DIRECTION ( 'NONE',  ( -1.000000000000000000, -0.000000000000000000, -0.000000000000000000 ) ) ;
#36017=CARTESIAN_POINT ( 'NONE',  ( 784.4999999999993179, -365.3551492539851893, -18.13243251470705886 ) ) ;
#36020=FACE_BOUND ( 'NONE', #5075, .T. ) ;
#36048=CARTESIAN_POINT ( 'NONE',  ( -26.63011601220122060, 26.27639943461401018, 900.0000000000001137 ) ) ;
#36059=PLANE ( 'NONE',  #26796 ) ;
#36081=EDGE_LOOP ( 'NONE', ( #30914, #42003, #45123, #12 ) ) ;
#36094=ORIENTED_EDGE ( 'NONE', *, *, #44162, .F. ) ;
#36107=VERTEX_POINT ( 'NONE', #23706 ) ;
#36126=ADVANCED_FACE ( 'NONE', ( #27198 ), #17252, .F. ) ;
#36130=AXIS2_PLACEMENT_3D ( 'NONE', #29514, #40977, #11511 ) ;
#36131=CARTESIAN_POINT ( 'NONE',  ( -26.63011601220122060, -544.8427095258973623, -350.0000000000000000 ) ) ;
#36139=CYLINDRICAL_SURFACE ( 'NONE', #39652, 19.99999999999990763 ) ;
#36141=EDGE_LOOP ( 'NONE', ( #19038, #1138, #6130, #14759, #44556, #4382 ) ) ;
#36179=DIRECTION ( 'NONE',  ( 0.000000000000000000, -0.3826834323650836756, -0.9238795325112892920 ) ) ;
#36192=ORIENTED_EDGE ( 'NONE', *, *, #32957, .F. ) ;
#36250=ORIENTED_EDGE ( 'NONE', *, *, #37961, .F. ) ;
#36268=EDGE_CURVE ( 'NONE', #1111, #9315, #9455, .T. ) ;
#36279=LINE ( 'NONE', #8124, #3089 ) ;
#36318=EDGE_CURVE ( 'NONE', #19003, #28399, #10103, .T. ) ;
#36322=ADVANCED_FACE ( 'NONE', ( #14941 ), #25559, .F. ) ;
#36350=DIRECTION ( 'NONE',  ( 0.000000000000000000, -0.6755902076156505842, -0.7372773368101328550 ) ) ;
#36358=CARTESIAN_POINT ( 'NONE',  ( -26.63011601220122060, -544.8427095258973623, -350.0000000000000000 ) ) ;
#36360=EDGE_LOOP ( 'NONE', ( #27232, #8824, #21598, #10029 ) ) ;
#36363=ORIENTED_EDGE ( 'NONE', *, *, #37672, .F. ) ;
#36374=DIRECTION ( 'NONE',  ( 0.000000000000000000, 0.000000000000000000, 1.000000000000000000 ) ) ;
#36378=CIRCLE ( 'NONE', #214, 19.99999999999990763 ) ;
#36382=CYLINDRICAL_SURFACE ( 'NONE', #24739, 9.999999999999980460 ) ;
#36393=CIRCLE ( 'NONE', #15007, 9.999999999999980460 ) ;
#36404=DIRECTION ( 'NONE',  ( -1.000000000000000000, -0.000000000000000000, -0.000000000000000000 ) ) ;
#36434=CARTESIAN_POINT ( 'NONE',  ( -39.63011601220123481, -513.1383975375929367, -369.9999999999999432 ) ) ;
#36436=DIRECTION ( 'NONE',  ( 1.000000000000000000, -0.000000000000000000, -0.000000000000000000 ) ) ;
#36452=ADVANCED_FACE ( 'NONE', ( #35486 ), #842, .T. ) ;
#36463=ORIENTED_EDGE ( 'NONE', *, *, #28665, .T. ) ;
#36465=VECTOR ( 'NONE', #43339, 1000.000000000000000 ) ;
#36501=DIRECTION ( 'NONE',  ( 0.000000000000000000, 0.3826834323650836200, 0.9238795325112892920 ) ) ;
#36511=CIRCLE ( 'NONE', #32093, 9.999999999999982236 ) ;
#36513=CARTESIAN_POINT ( 'NONE',  ( -786.4999999999993179, 262.9227088301245203, 634.7515695135432452 ) ) ;
#36529=EDGE_CURVE ( 'NONE', #463, #45642, #43340, .T. ) ;
#36530=VECTOR ( 'NONE', #22956, 1000.000000000000000 ) ;
#36535=VERTEX_POINT ( 'NONE', #14726 ) ;
#36538=ADVANCED_FACE ( 'NONE', ( #24867 ), #25780, .F. ) ;
#36546=AXIS2_PLACEMENT_3D ( 'NONE', #5872, #32996, #27124 ) ;
#36555=DIRECTION ( 'NONE',  ( -1.000000000000000000, -0.000000000000000000, -0.000000000000000000 ) ) ;
#36560=AXIS2_PLACEMENT_3D ( 'NONE', #24295, #38401, #6751 ) ;
#36561=DIRECTION ( 'NONE',  ( -0.000000000000000000, -0.3826834323650836756, -0.9238795325112892920 ) ) ;
#36564=EDGE_CURVE ( 'NONE', #41202, #20268, #44899, .T. ) ;
#36592=UNCERTAINTY_MEASURE_WITH_UNIT (LENGTH_MEASURE( 1.000000000000000082E-05 ), #43968, 'distance_accuracy_value', 'NONE');
#36596=ORIENTED_EDGE ( 'NONE', *, *, #6009, .T. ) ;
#36605=ORIENTED_EDGE ( 'NONE', *, *, #4428, .F. ) ;
#36607=EDGE_LOOP ( 'NONE', ( #32223, #5577, #16252, #14228 ) ) ;
#36647=ORIENTED_EDGE ( 'NONE', *, *, #15570, .T. ) ;
#36666=PLANE ( 'NONE',  #9251 ) ;
#36693=CARTESIAN_POINT ( 'NONE',  ( -39.63011601220123481, -512.9681489794448908, -329.9999999999999432 ) ) ;
#36715=ORIENTED_EDGE ( 'NONE', *, *, #30000, .T. ) ;
#36723=PLANE ( 'NONE',  #1238 ) ;
#36764=VERTEX_POINT ( 'NONE', #11245 ) ;
#36781=VERTEX_POINT ( 'NONE', #3642 ) ;
#36785=DIRECTION ( 'NONE',  ( 0.000000000000000000, 0.000000000000000000, 1.000000000000000000 ) ) ;
#36793=DIRECTION ( 'NONE',  ( 0.000000000000000000, -0.9238795325112891810, 0.3826834323650837866 ) ) ;
#36807=ORIENTED_EDGE ( 'NONE', *, *, #2367, .T. ) ;
#36851=VECTOR ( 'NONE', #3561, 1000.000000000000000 ) ;
#36857=CARTESIAN_POINT ( 'NONE',  ( -26.63011601220122060, -513.1383975375929367, -369.9999999999999432 ) ) ;
#36863=LINE ( 'NONE', #2426, #18110 ) ;
#36874=EDGE_CURVE ( 'NONE', #9279, #5066, #19832, .T. ) ;
#36920=VERTEX_POINT ( 'NONE', #5836 ) ;
#36952=FACE_BOUND ( 'NONE', #42278, .T. ) ;
#36975=DIRECTION ( 'NONE',  ( 1.000000000000000000, 0.000000000000000000, -0.000000000000000000 ) ) ;
#36987=ORIENTED_EDGE ( 'NONE', *, *, #26462, .F. ) ;
#36992=CARTESIAN_POINT ( 'NONE',  ( -773.4999999999993179, -494.6608068873671300, -357.6536686473015720 ) ) ;
#36999=CARTESIAN_POINT ( 'NONE',  ( -26.63011601220122060, -110.5936016518799221, 750.6326042729449455 ) ) ;
#37001=APPLICATION_CONTEXT ( 'automotive_design' ) ;
#37007=CIRCLE ( 'NONE', #28919, 19.99999999999990763 ) ;
#37017=CARTESIAN_POINT ( 'NONE',  ( 786.4999999999993179, -512.9681489794448908, -327.9999999999999432 ) ) ;
#37024=UNCERTAINTY_MEASURE_WITH_UNIT (LENGTH_MEASURE( 1.000000000000000082E-05 ), #32820, 'distance_accuracy_value', 'NONE');
#37029=EDGE_LOOP ( 'NONE', ( #18666, #3768, #11037, #37261 ) ) ;
#37035=VECTOR ( 'NONE', #15596, 1000.000000000000114 ) ;
#37041=DIRECTION ( 'NONE',  ( 1.000000000000000000, 0.000000000000000000, -0.000000000000000000 ) ) ;
#37065=EDGE_CURVE ( 'NONE', #2171, #36781, #2856, .T. ) ;
#37076=DIRECTION ( 'NONE',  ( -0.000000000000000000, -0.6755902076156505842, -0.7372773368101327440 ) ) ;
#37106=CARTESIAN_POINT ( 'NONE',  ( -28.63011601220122415, -544.8427095258973623, -369.9999999999999432 ) ) ;
#37117=ADVANCED_FACE ( 'NONE', ( #42300 ), #10664, .T. ) ;
#37141=EDGE_CURVE ( 'NONE', #9315, #17287, #21289, .T. ) ;
#37143=LINE ( 'NONE', #37384, #37201 ) ;
#37144=ORIENTED_EDGE ( 'NONE', *, *, #15665, .F. ) ;
#37152=CIRCLE ( 'NONE', #17254, 20.00000000000001776 ) ;
#37154=VECTOR ( 'NONE', #17884, 1000.000000000000114 ) ;
#37160=DIRECTION ( 'NONE',  ( 0.000000000000000000, 0.000000000000000000, -1.000000000000000000 ) ) ;
#37185=CIRCLE ( 'NONE', #17285, 9.999999999999982236 ) ;
#37198=VERTEX_POINT ( 'NONE', #20595 ) ;
#37201=VECTOR ( 'NONE', #1800, 1000.000000000000114 ) ;
#37220=ORIENTED_EDGE ( 'NONE', *, *, #10099, .T. ) ;
#37224=DIRECTION ( 'NONE',  ( 0.000000000000000000, 0.000000000000000000, -1.000000000000000000 ) ) ;
#37240=AXIS2_PLACEMENT_3D ( 'NONE', #21041, #34680, #19741 ) ;
#37246=CARTESIAN_POINT ( 'NONE',  ( -39.63011601220123481, 26.27639943461401018, 900.0000000000001137 ) ) ;
#37261=ORIENTED_EDGE ( 'NONE', *, *, #28090, .T. ) ;
#37265=ORIENTED_EDGE ( 'NONE', *, *, #7148, .F. ) ;
#37268=VERTEX_POINT ( 'NONE', #38613 ) ;
#37277=ORIENTED_EDGE ( 'NONE', *, *, #19836, .F. ) ;
#37281=VERTEX_POINT ( 'NONE', #3741 ) ;
#37316=VECTOR ( 'NONE', #15374, 1000.000000000000000 ) ;
#37379=ORIENTED_EDGE ( 'NONE', *, *, #15407, .T. ) ;
#37384=CARTESIAN_POINT ( 'NONE',  ( 775.4999999999993179, -501.1515549466498669, -368.0974687824633520 ) ) ;
#37385=EDGE_CURVE ( 'NONE', #37268, #23506, #35589, .T. ) ;
#37389=EDGE_CURVE ( 'NONE', #40120, #13363, #35296, .T. ) ;
#37397=ORIENTED_EDGE ( 'NONE', *, *, #37429, .F. ) ;
#37429=EDGE_CURVE ( 'NONE', #8747, #34761, #42763, .T. ) ;
#37441=CARTESIAN_POINT ( 'NONE',  ( 786.4999999999993179, -434.0043448692482002, 397.6917108626901154 ) ) ;
#37442=ORIENTED_EDGE ( 'NONE', *, *, #19077, .T. ) ;
#37451=ORIENTED_EDGE ( 'NONE', *, *, #5821, .F. ) ;
#37459=LINE ( 'NONE', #31204, #9362 ) ;
#37471=FACE_OUTER_BOUND ( 'NONE', #18770, .T. ) ;
#37497=( NAMED_UNIT ( * ) PLANE_ANGLE_UNIT ( ) SI_UNIT ( $, .RADIAN. ) );
#37500=ORIENTED_EDGE ( 'NONE', *, *, #15904, .F. ) ;
#37508=FACE_OUTER_BOUND ( 'NONE', #5337, .T. ) ;
#37526=DIRECTION ( 'NONE',  ( 0.000000000000000000, 0.000000000000000000, 1.000000000000000000 ) ) ;
#37580=EDGE_CURVE ( 'NONE', #7814, #24322, #39014, .T. ) ;
#37597=EDGE_CURVE ( 'NONE', #41202, #32812, #39306, .T. ) ;
#37599=DIRECTION ( 'NONE',  ( -0.000000000000000000, -0.3826834323650838976, -0.9238795325112892920 ) ) ;
#37672=EDGE_CURVE ( 'NONE', #10339, #29708, #27973, .T. ) ;
#37679=ORIENTED_EDGE ( 'NONE', *, *, #32011, .T. ) ;
#37700=DIRECTION ( 'NONE',  ( 0.000000000000000000, 0.000000000000000000, -1.000000000000000000 ) ) ;
#37735=CARTESIAN_POINT ( 'NONE',  ( 784.4999999999993179, -355.4967352946684969, -16.45562775363623587 ) ) ;
#37742=ORIENTED_EDGE ( 'NONE', *, *, #28090, .F. ) ;
#37744=VECTOR ( 'NONE', #14603, 1000.000000000000227 ) ;
#37749=CIRCLE ( 'NONE', #34808, 9.999999999999982236 ) ;
#37751=CARTESIAN_POINT ( 'NONE',  ( -28.63011601220122415, -513.1383975375929367, -367.9999999999999432 ) ) ;
#37756=DIRECTION ( 'NONE',  ( -1.000000000000000000, 0.000000000000000000, 0.000000000000000000 ) ) ;
#37766=DIRECTION ( 'NONE',  ( 1.000000000000000000, 0.000000000000000000, -0.000000000000000000 ) ) ;
#37782=ORIENTED_EDGE ( 'NONE', *, *, #21258, .F. ) ;
#37808=CARTESIAN_POINT ( 'NONE',  ( -786.4999999999993179, 26.27639943461401018, 900.0000000000001137 ) ) ;
#37811=VERTEX_POINT ( 'NONE', #15720 ) ;
#37828=EDGE_LOOP ( 'NONE', ( #22771, #26415, #14119, #33573 ) ) ;
#37855=LINE ( 'NONE', #26761, #39363 ) ;
#37863=PRODUCT_DEFINITION_FORMATION_WITH_SPECIFIED_SOURCE ( 'ANY', '', #38425, .NOT_KNOWN. ) ;
#37885=DIRECTION ( 'NONE',  ( 0.000000000000000000, 0.000000000000000000, 1.000000000000000000 ) ) ;
#37895=VECTOR ( 'NONE', #8690, 1000.000000000000114 ) ;
#37908=VECTOR ( 'NONE', #20186, 1000.000000000000114 ) ;
#37937=CARTESIAN_POINT ( 'NONE',  ( -37.63011601220122770, -513.1383975375929367, -350.0000000000000000 ) ) ;
#37946=AXIS2_PLACEMENT_3D ( 'NONE', #36857, #40096, #44238 ) ;
#37954=ORIENTED_EDGE ( 'NONE', *, *, #42697, .F. ) ;
#37961=EDGE_CURVE ( 'NONE', #34249, #10339, #5782, .T. ) ;
#37969=CARTESIAN_POINT ( 'NONE',  ( -28.63011601220122415, -544.8427095258973623, -369.9999999999999432 ) ) ;
#37972=CARTESIAN_POINT ( 'NONE',  ( 786.4999999999993179, -110.5936016518798652, 750.6326042729449455 ) ) ;
#38033=LINE ( 'NONE', #27178, #18151 ) ;
#38055=CARTESIAN_POINT ( 'NONE',  ( 786.4999999999993179, -110.5936016518799221, 750.6326042729449455 ) ) ;
#38057=DIRECTION ( 'NONE',  ( 0.000000000000000000, 0.000000000000000000, -1.000000000000000000 ) ) ;
#38068=EDGE_CURVE ( 'NONE', #24322, #42149, #12482, .T. ) ;
#38085=AXIS2_PLACEMENT_3D ( 'NONE', #2388, #9336, #24952 ) ;
#38112=VECTOR ( 'NONE', #40811, 1000.000000000000000 ) ;
#38166=CARTESIAN_POINT ( 'NONE',  ( 775.4999999999993179, -365.3551492539851893, -18.13243251470705886 ) ) ;
#38172=CARTESIAN_POINT ( 'NONE',  ( -775.4999999999993179, -359.5698779088871788, -26.28906389436296109 ) ) ;
#38191=VERTEX_POINT ( 'NONE', #27029 ) ;
#38263=LINE ( 'NONE', #13096, #2614 ) ;
#38275=LINE ( 'NONE', #40085, #38533 ) ;
#38276=DIRECTION ( 'NONE',  ( -1.000000000000000000, -0.000000000000000000, 0.000000000000000000 ) ) ;
#38277=EDGE_CURVE ( 'NONE', #4067, #36764, #23997, .T. ) ;
#38288=ORIENTED_EDGE ( 'NONE', *, *, #33206, .T. ) ;
#38295=EDGE_CURVE ( 'NONE', #12731, #40960, #2892, .T. ) ;
#38308=VECTOR ( 'NONE', #17782, 1000.000000000000000 ) ;
#38377=DIRECTION ( 'NONE',  ( 0.000000000000000000, 0.9238795325112891810, -0.3826834323650838421 ) ) ;
#38382=LINE ( 'NONE', #34903, #21516 ) ;
#38401=DIRECTION ( 'NONE',  ( 1.000000000000000000, 0.000000000000000000, -0.000000000000000000 ) ) ;
#38425=PRODUCT ( 'Foot Treadle Lever Assembly', 'Foot Treadle Lever Assembly', '', ( #24650 ) ) ;
#38436=FACE_BOUND ( 'NONE', #2175, .T. ) ;
#38442=( NAMED_UNIT ( * ) SI_UNIT ( $, .STERADIAN. ) SOLID_ANGLE_UNIT ( ) );
#38453=CARTESIAN_POINT ( 'NONE',  ( -33.13011601220117086, -513.1383975375929367, -367.9999999999999432 ) ) ;
#38485=DIRECTION ( 'NONE',  ( 0.000000000000000000, 0.000000000000000000, 1.000000000000000000 ) ) ;
#38495=CYLINDRICAL_SURFACE ( 'NONE', #21675, 10.00000000000000888 ) ;
#38498=DIRECTION ( 'NONE',  ( 0.000000000000000000, 0.000000000000000000, 1.000000000000000000 ) ) ;
#38519=ADVANCED_FACE ( 'NONE', ( #25352 ), #11276, .F. ) ;
#38533=VECTOR ( 'NONE', #42650, 1000.000000000000227 ) ;
#38542=CARTESIAN_POINT ( 'NONE',  ( -786.4999999999993179, -494.6608068873671300, -357.6536686473015720 ) ) ;
#38546=VERTEX_POINT ( 'NONE', #4571 ) ;
#38550=CARTESIAN_POINT ( 'NONE',  ( -784.4999999999993179, -544.8427095258973623, -350.0000000000000000 ) ) ;
#38559=ADVANCED_FACE ( 'NONE', ( #11742 ), #26022, .T. ) ;
#38567=ADVANCED_FACE ( 'NONE', ( #18662 ), #42909, .F. ) ;
#38589=AXIS2_PLACEMENT_3D ( 'NONE', #25307, #43757, #32482 ) ;
#38594=CARTESIAN_POINT ( 'NONE',  ( -39.63011601220123481, -512.9681489794448908, -350.0000000000000000 ) ) ;
#38613=CARTESIAN_POINT ( 'NONE',  ( 775.4999999999993179, -544.8427095258973623, -369.9999999999999432 ) ) ;
#38657=LINE ( 'NONE', #34952, #32897 ) ;
#38658=CYLINDRICAL_SURFACE ( 'NONE', #1203, 19.99999999999990763 ) ;
#38675=DIRECTION ( 'NONE',  ( 0.000000000000000000, 1.000000000000000000, -0.000000000000000000 ) ) ;
#38688=LINE ( 'NONE', #38453, #20297 ) ;
#38693=VECTOR ( 'NONE', #25238, 1000.000000000000000 ) ;
#38697=DIRECTION ( 'NONE',  ( 0.000000000000000000, -0.3826834323650836756, -0.9238795325112892920 ) ) ;
#38730=CLOSED_SHELL ( 'NONE', ( #32894, #33738, #3550, #26305, #4169, #34654, #42769, #10019, #6065, #23504, #21622, #34601, #44733, #15446, #22501, #28053, #9698, #34239, #5518, #7393, #4398, #38559, #44784, #19850 ) ) ;
#38780=AXIS2_PLACEMENT_3D ( 'NONE', #43406, #6987, #32557 ) ;
#38781=LINE ( 'NONE', #197, #31448 ) ;
#38798=EDGE_CURVE ( 'NONE', #757, #30488, #20177, .T. ) ;
#38802=( LENGTH_UNIT ( ) NAMED_UNIT ( * ) SI_UNIT ( .MILLI., .METRE. ) );
#38862=DIRECTION ( 'NONE',  ( 0.000000000000000000, 0.000000000000000000, 1.000000000000000000 ) ) ;
#38897=ORIENTED_EDGE ( 'NONE', *, *, #31530, .T. ) ;
#38919=DIRECTION ( 'NONE',  ( 0.000000000000000000, -0.6755902076156404812, -0.7372773368101421809 ) ) ;
#38945=ORIENTED_EDGE ( 'NONE', *, *, #10584, .F. ) ;
#38954=VERTEX_POINT ( 'NONE', #37969 ) ;
#38972=DIRECTION ( 'NONE',  ( 0.000000000000000000, 0.000000000000000000, 1.000000000000000000 ) ) ;
#38977=DIRECTION ( 'NONE',  ( 0.000000000000000000, 0.000000000000000000, 1.000000000000000000 ) ) ;
#38984=DIRECTION ( 'NONE',  ( -1.000000000000000000, -0.000000000000000000, 0.000000000000000000 ) ) ;
#38993=CARTESIAN_POINT ( 'NONE',  ( -786.4999999999993179, -365.3551492539851893, -18.13243251470705886 ) ) ;
#39002=ORIENTED_EDGE ( 'NONE', *, *, #3532, .F. ) ;
#39014=CIRCLE ( 'NONE', #13221, 19.99999999999990763 ) ;
#39030=EDGE_CURVE ( 'NONE', #17123, #42371, #34723, .T. ) ;
#39033=CARTESIAN_POINT ( 'NONE',  ( 773.4999999999993179, 26.27639943461401018, 900.0000000000001137 ) ) ;
#39046=VECTOR ( 'NONE', #26560, 1000.000000000000000 ) ;
#39064=VERTEX_POINT ( 'NONE', #31495 ) ;
#39109=ORIENTED_EDGE ( 'NONE', *, *, #14545, .F. ) ;
#39128=CARTESIAN_POINT ( 'NONE',  ( 775.4999999999993179, -544.8427095258973623, -350.0000000000000000 ) ) ;
#39148=LINE ( 'NONE', #31524, #29864 ) ;
#39155=DIRECTION ( 'NONE',  ( 1.000000000000000000, 0.000000000000000000, -0.000000000000000000 ) ) ;
#39183=ORIENTED_EDGE ( 'NONE', *, *, #33660, .T. ) ;
#39205=CARTESIAN_POINT ( 'NONE',  ( -746.4999999999993179, -359.5698779088871788, -26.28906389436294688 ) ) ;
#39212=VERTEX_POINT ( 'NONE', #77 ) ;
#39222=ADVANCED_BREP_SHAPE_REPRESENTATION ( '', ( #1418, #33391, #17697, #3320, #26858 ), #34210 ) ;
#39241=CARTESIAN_POINT ( 'NONE',  ( -786.4999999999993179, 26.27639943461401018, 900.0000000000001137 ) ) ;
#39246=VECTOR ( 'NONE', #21046, 1000.000000000000000 ) ;
#39253=( NAMED_UNIT ( * ) PLANE_ANGLE_UNIT ( ) SI_UNIT ( $, .RADIAN. ) );
#39306=LINE ( 'NONE', #43666, #8798 ) ;
#39331=ORIENTED_EDGE ( 'NONE', *, *, #12847, .F. ) ;
#39344=LINE ( 'NONE', #4467, #34395 ) ;
#39353=DIRECTION ( 'NONE',  ( 0.000000000000000000, 0.3826834323650836756, 0.9238795325112892920 ) ) ;
#39358=CIRCLE ( 'NONE', #19422, 12.00000000000001066 ) ;
#39363=VECTOR ( 'NONE', #9904, 1000.000000000000000 ) ;
#39374=CYLINDRICAL_SURFACE ( 'NONE', #23258, 20.00000000000001776 ) ;
#39385=DIRECTION ( 'NONE',  ( 0.000000000000000000, 0.000000000000000000, 1.000000000000000000 ) ) ;
#39412=DIRECTION ( 'NONE',  ( -1.000000000000000000, -0.000000000000000000, 0.000000000000000000 ) ) ;
#39466=DIRECTION ( 'NONE',  ( 0.000000000000000000, 0.7372773368101328550, -0.6755902076156506952 ) ) ;
#39470=EDGE_LOOP ( 'NONE', ( #22553, #14769, #28863, #9454 ) ) ;
#39514=VECTOR ( 'NONE', #385, 999.9999999999998863 ) ;
#39516=CARTESIAN_POINT ( 'NONE',  ( 786.4999999999993179, -110.5936016518799221, 750.6326042729449455 ) ) ;
#39517=VERTEX_POINT ( 'NONE', #8379 ) ;
#39543=CARTESIAN_POINT ( 'NONE',  ( -39.63011601220123481, -544.8427095258973623, -350.0000000000000000 ) ) ;
#39547=VECTOR ( 'NONE', #32002, 1000.000000000000000 ) ;
#39612=ORIENTED_EDGE ( 'NONE', *, *, #19077, .F. ) ;
#39618=DIRECTION ( 'NONE',  ( 0.000000000000000000, 0.3826834323650838421, 0.9238795325112891810 ) ) ;
#39635=ORIENTED_EDGE ( 'NONE', *, *, #5821, .T. ) ;
#39647=VERTEX_POINT ( 'NONE', #36992 ) ;
#39652=AXIS2_PLACEMENT_3D ( 'NONE', #11427, #42839, #39385 ) ;
#39678=DIRECTION ( 'NONE',  ( 1.000000000000000000, -0.000000000000000000, -0.000000000000000000 ) ) ;
#39689=VECTOR ( 'NONE', #44599, 1000.000000000000000 ) ;
#39697=VERTEX_POINT ( 'NONE', #32869 ) ;
#39713=LINE ( 'NONE', #29519, #35899 ) ;
#39739=DIRECTION ( 'NONE',  ( 0.000000000000000000, -0.6755902076156505842, -0.7372773368101327440 ) ) ;
#39752=ADVANCED_FACE ( 'NONE', ( #5134 ), #44153, .F. ) ;
#39774=DIRECTION ( 'NONE',  ( 0.000000000000000000, 0.000000000000000000, -1.000000000000000000 ) ) ;
#39800=CARTESIAN_POINT ( 'NONE',  ( 773.4999999999993179, 26.27639943461401018, 900.0000000000001137 ) ) ;
#39819=FACE_OUTER_BOUND ( 'NONE', #9867, .T. ) ;
#39855=ORIENTED_EDGE ( 'NONE', *, *, #25795, .T. ) ;
#39861=ORIENTED_EDGE ( 'NONE', *, *, #31530, .F. ) ;
#39870=ORIENTED_EDGE ( 'NONE', *, *, #39951, .T. ) ;
#39881=PLANE ( 'NONE',  #10526 ) ;
#39896=FACE_OUTER_BOUND ( 'NONE', #10630, .T. ) ;
#39900=EDGE_CURVE ( 'NONE', #44015, #16954, #37459, .T. ) ;
#39907=ORIENTED_EDGE ( 'NONE', *, *, #14562, .F. ) ;
#39951=EDGE_CURVE ( 'NONE', #17108, #22668, #44853, .T. ) ;
#39959=CARTESIAN_POINT ( 'NONE',  ( 775.4999999999993179, -513.1383975375929367, -369.9999999999999432 ) ) ;
#40009=CARTESIAN_POINT ( 'NONE',  ( -26.63011601220122060, -512.9681489794448908, -350.0000000000000000 ) ) ;
#40010=VERTEX_POINT ( 'NONE', #6032 ) ;
#40032=DIRECTION ( 'NONE',  ( 1.000000000000000000, 0.000000000000000000, -0.000000000000000000 ) ) ;
#40085=CARTESIAN_POINT ( 'NONE',  ( -26.63011601220122060, -494.6608068873671300, -357.6536686473015720 ) ) ;
#40089=CARTESIAN_POINT ( 'NONE',  ( -26.63011601220122060, -496.5085659523897448, -356.8883017825714319 ) ) ;
#40091=VECTOR ( 'NONE', #17688, 1000.000000000000114 ) ;
#40096=DIRECTION ( 'NONE',  ( 0.000000000000000000, 1.000000000000000000, -0.000000000000000000 ) ) ;
#40102=DIRECTION ( 'NONE',  ( -1.000000000000000000, -0.000000000000000000, -0.000000000000000000 ) ) ;
#40120=VERTEX_POINT ( 'NONE', #24264 ) ;
#40128=CARTESIAN_POINT ( 'NONE',  ( -786.4999999999993179, -30.07539427629363260, 756.1153575698151599 ) ) ;
#40161=VERTEX_POINT ( 'NONE', #13435 ) ;
#40166=CARTESIAN_POINT ( 'NONE',  ( -784.4999999999993179, -563.3203001761230553, -342.3463313526983143 ) ) ;
#40181=EDGE_CURVE ( 'NONE', #22673, #19543, #16676, .T. ) ;
#40240=PLANE ( 'NONE',  #33752 ) ;
#40241=ORIENTED_EDGE ( 'NONE', *, *, #45565, .F. ) ;
#40254=VECTOR ( 'NONE', #17760, 1000.000000000000000 ) ;
#40273=VECTOR ( 'NONE', #17007, 1000.000000000000000 ) ;
#40283=DIRECTION ( 'NONE',  ( -1.000000000000000000, -0.000000000000000000, -0.000000000000000000 ) ) ;
#40284=ORIENTED_EDGE ( 'NONE', *, *, #23827, .T. ) ;
#40288=AXIS2_PLACEMENT_3D ( 'NONE', #34722, #16488, #17414 ) ;
#40289=CARTESIAN_POINT ( 'NONE',  ( -37.63011601220122770, -365.3551492539851893, -8.132432514707076621 ) ) ;
#40293=ORIENTED_EDGE ( 'NONE', *, *, #9416, .F. ) ;
#40307=AXIS2_PLACEMENT_3D ( 'NONE', #247, #23406, #34031 ) ;
#40310=VERTEX_POINT ( 'NONE', #38594 ) ;
#40334=VECTOR ( 'NONE', #17176, 1000.000000000000000 ) ;
#40357=( LENGTH_UNIT ( ) NAMED_UNIT ( * ) SI_UNIT ( .MILLI., .METRE. ) );
#40369=EDGE_LOOP ( 'NONE', ( #35168, #17393, #32176, #18927, #21960, #12341 ) ) ;
#40383=DIRECTION ( 'NONE',  ( 0.000000000000000000, 0.000000000000000000, -1.000000000000000000 ) ) ;
#40391=CARTESIAN_POINT ( 'NONE',  ( 775.4999999999993179, -512.9681489794448908, -339.9999999999999432 ) ) ;
#40396=ORIENTED_EDGE ( 'NONE', *, *, #37597, .F. ) ;
#40407=FACE_OUTER_BOUND ( 'NONE', #33015, .T. ) ;
#40415=ORIENTED_EDGE ( 'NONE', *, *, #28049, .F. ) ;
#40422=ORIENTED_EDGE ( 'NONE', *, *, #4401, .F. ) ;
#40429=DIRECTION ( 'NONE',  ( -1.000000000000000000, -0.000000000000000000, -0.000000000000000000 ) ) ;
#40487=PLANE ( 'NONE',  #5450 ) ;
#40494=FACE_OUTER_BOUND ( 'NONE', #36360, .T. ) ;
#40510=EDGE_CURVE ( 'NONE', #29224, #2171, #21719, .T. ) ;
#40525=ORIENTED_EDGE ( 'NONE', *, *, #15904, .T. ) ;
#40528=EDGE_CURVE ( 'NONE', #37281, #7806, #1705, .T. ) ;
#40597=CARTESIAN_POINT ( 'NONE',  ( -775.4999999999993179, -501.1515549466498669, -368.0974687824633520 ) ) ;
#40606=LINE ( 'NONE', #32379, #9232 ) ;
#40618=DIRECTION ( 'NONE',  ( -0.000000000000000000, 0.000000000000000000, 1.000000000000000000 ) ) ;
#40621=VERTEX_POINT ( 'NONE', #33711 ) ;
#40699=CARTESIAN_POINT ( 'NONE',  ( 775.4999999999993179, -359.5698779088871788, -26.28906389436296109 ) ) ;
#40741=ADVANCED_FACE ( 'NONE', ( #8559 ), #8994, .F. ) ;
#40744=DIRECTION ( 'NONE',  ( 1.000000000000000000, 0.000000000000000000, 0.000000000000000000 ) ) ;
#40751=DIRECTION ( 'NONE',  ( 0.000000000000000000, 0.000000000000000000, 1.000000000000000000 ) ) ;
#40764=LINE ( 'NONE', #41000, #45283 ) ;
#40777=CARTESIAN_POINT ( 'NONE',  ( -775.4999999999993179, -857.0166862835568509, -63.94525337997358605 ) ) ;
#40785=LINE ( 'NONE', #22776, #34160 ) ;
#40794=ORIENTED_EDGE ( 'NONE', *, *, #26985, .T. ) ;
#40804=EDGE_CURVE ( 'NONE', #16495, #34761, #43427, .T. ) ;
#40811=DIRECTION ( 'NONE',  ( 0.000000000000000000, 1.000000000000000000, -0.000000000000000000 ) ) ;
#40842=ORIENTED_EDGE ( 'NONE', *, *, #29773, .F. ) ;
#40870=ORIENTED_EDGE ( 'NONE', *, *, #40510, .F. ) ;
#40894=FACE_OUTER_BOUND ( 'NONE', #31579, .T. ) ;
#40905=AXIS2_PLACEMENT_3D ( 'NONE', #45454, #34357, #6641 ) ;
#40908=CIRCLE ( 'NONE', #2526, 19.99999999999990763 ) ;
#40949=CARTESIAN_POINT ( 'NONE',  ( -786.4999999999993179, -110.5936016518798652, 750.6326042729449455 ) ) ;
#40953=ORIENTED_EDGE ( 'NONE', *, *, #11738, .F. ) ;
#40960=VERTEX_POINT ( 'NONE', #23743 ) ;
#40977=DIRECTION ( 'NONE',  ( 0.000000000000000000, -0.9238795325112892920, 0.3826834323650836756 ) ) ;
#41000=CARTESIAN_POINT ( 'NONE',  ( -26.63011601220122060, -513.1383975375929367, -369.9999999999999432 ) ) ;
#41026=EDGE_CURVE ( 'NONE', #40960, #7806, #37855, .T. ) ;
#41044=LINE ( 'NONE', #20017, #38112 ) ;
#41061=ORIENTED_EDGE ( 'NONE', *, *, #21315, .T. ) ;
#41084=AXIS2_PLACEMENT_3D ( 'NONE', #11958, #36436, #26026 ) ;
#41089=ORIENTED_EDGE ( 'NONE', *, *, #29222, .F. ) ;
#41109=VERTEX_POINT ( 'NONE', #3201 ) ;
#41146=ORIENTED_EDGE ( 'NONE', *, *, #21098, .T. ) ;
#41172=FACE_OUTER_BOUND ( 'NONE', #26727, .T. ) ;
#41202=VERTEX_POINT ( 'NONE', #34626 ) ;
#41210=FACE_BOUND ( 'NONE', #43196, .T. ) ;
#41212=CARTESIAN_POINT ( 'NONE',  ( 746.4999999999993179, -359.5698779088871788, -26.28906389436294688 ) ) ;
#41227=DIRECTION ( 'NONE',  ( -1.000000000000000000, -0.000000000000000000, -0.000000000000000000 ) ) ;
#41230=CARTESIAN_POINT ( 'NONE',  ( -786.4999999999993179, -563.3203001761230553, -342.3463313526983143 ) ) ;
#41269=VECTOR ( 'NONE', #10544, 1000.000000000000000 ) ;
#41294=EDGE_CURVE ( 'NONE', #15262, #11223, #18234, .T. ) ;
#41302=ORIENTED_EDGE ( 'NONE', *, *, #15175, .F. ) ;
#41421=EDGE_LOOP ( 'NONE', ( #4667, #37742, #11992, #31249, #7686, #3312, #27003, #24353, #13932, #8555, #41089 ) ) ;
#41489=DIRECTION ( 'NONE',  ( -1.000000000000000000, -0.000000000000000000, 0.000000000000000000 ) ) ;
#41500=LINE ( 'NONE', #45192, #41741 ) ;
#41530=EDGE_LOOP ( 'NONE', ( #19584, #42050, #26645, #23727, #9410, #28068, #14054, #25339, #17274, #19490, #20120 ) ) ;
#41585=EDGE_CURVE ( 'NONE', #4358, #14962, #7836, .T. ) ;
#41602=CIRCLE ( 'NONE', #9123, 9.999999999999980460 ) ;
#41613=EDGE_CURVE ( 'NONE', #43251, #39517, #4580, .T. ) ;
#41622=CARTESIAN_POINT ( 'NONE',  ( 784.4999999999993179, -512.9681489794448908, -339.9999999999999432 ) ) ;
#41649=ORIENTED_EDGE ( 'NONE', *, *, #36318, .F. ) ;
#41656=VECTOR ( 'NONE', #44637, 1000.000000000000000 ) ;
#41671=ORIENTED_EDGE ( 'NONE', *, *, #23841, .F. ) ;
#41710=LINE ( 'NONE', #3601, #40091 ) ;
#41718=VECTOR ( 'NONE', #13923, 1000.000000000000000 ) ;
#41741=VECTOR ( 'NONE', #31774, 1000.000000000000000 ) ;
#41749=CIRCLE ( 'NONE', #26993, 9.999999999999982236 ) ;
#41769=AXIS2_PLACEMENT_3D ( 'NONE', #5868, #29893, #16260 ) ;
#41795=ORIENTED_EDGE ( 'NONE', *, *, #32094, .T. ) ;
#41806=VECTOR ( 'NONE', #5927, 1000.000000000000000 ) ;
#41823=ORIENTED_EDGE ( 'NONE', *, *, #40181, .T. ) ;
#41849=CARTESIAN_POINT ( 'NONE',  ( 786.4999999999993179, -110.5936016518799221, 750.6326042729449455 ) ) ;
#41861=CARTESIAN_POINT ( 'NONE',  ( 786.4999999999993179, -512.9681489794448908, -329.9999999999999432 ) ) ;
#41882=LINE ( 'NONE', #13704, #16818 ) ;
#41886=EDGE_LOOP ( 'NONE', ( #11108, #41061, #30017, #24245 ) ) ;
#41900=CARTESIAN_POINT ( 'NONE',  ( -28.63011601220122415, -365.3551492539851893, -18.13243251470705886 ) ) ;
#41907=EDGE_CURVE ( 'NONE', #26595, #12779, #15651, .T. ) ;
#41917=LINE ( 'NONE', #20648, #37154 ) ;
#41918=DIRECTION ( 'NONE',  ( 1.000000000000000000, -0.000000000000000000, -0.000000000000000000 ) ) ;
#41934=ORIENTED_EDGE ( 'NONE', *, *, #6964, .T. ) ;
#41991=ORIENTED_EDGE ( 'NONE', *, *, #6908, .T. ) ;
#42003=ORIENTED_EDGE ( 'NONE', *, *, #33200, .F. ) ;
#42024=FACE_BOUND ( 'NONE', #32924, .T. ) ;
#42050=ORIENTED_EDGE ( 'NONE', *, *, #7810, .T. ) ;
#42067=PLANE ( 'NONE',  #37240 ) ;
#42114=EDGE_CURVE ( 'NONE', #44996, #44015, #12637, .T. ) ;
#42130=FACE_OUTER_BOUND ( 'NONE', #28022, .T. ) ;
#42133=CYLINDRICAL_SURFACE ( 'NONE', #2505, 10.00000000000000888 ) ;
#42149=VERTEX_POINT ( 'NONE', #34337 ) ;
#42196=CARTESIAN_POINT ( 'NONE',  ( 786.4999999999993179, -496.5085659523897448, -356.8883017825714319 ) ) ;
#42205=CARTESIAN_POINT ( 'NONE',  ( -775.4999999999993179, -365.3551492539851893, -18.13243251470705886 ) ) ;
#42209=CARTESIAN_POINT ( 'NONE',  ( -786.4999999999993179, -365.3551492539851893, -28.13243251470704109 ) ) ;
#42278=EDGE_LOOP ( 'NONE', ( #9077, #1795 ) ) ;
#42280=FACE_OUTER_BOUND ( 'NONE', #4851, .T. ) ;
#42296=DIRECTION ( 'NONE',  ( -0.000000000000000000, 1.000000000000000000, -0.000000000000000000 ) ) ;
#42300=FACE_OUTER_BOUND ( 'NONE', #11715, .T. ) ;
#42321=FACE_OUTER_BOUND ( 'NONE', #29882, .T. ) ;
#42330=ORIENTED_EDGE ( 'NONE', *, *, #8660, .T. ) ;
#42334=CARTESIAN_POINT ( 'NONE',  ( -28.63011601220122415, -544.8427095258973623, -350.0000000000000000 ) ) ;
#42351=LINE ( 'NONE', #45615, #14479 ) ;
#42367=FACE_OUTER_BOUND ( 'NONE', #36141, .T. ) ;
#42371=VERTEX_POINT ( 'NONE', #16330 ) ;
#42387=VERTEX_POINT ( 'NONE', #30412 ) ;
#42397=ORIENTED_EDGE ( 'NONE', *, *, #28049, .T. ) ;
#42407=CARTESIAN_POINT ( 'NONE',  ( 773.4999999999993179, -544.8427095258973623, -350.0000000000000000 ) ) ;
#42442=VECTOR ( 'NONE', #7382, 1000.000000000000114 ) ;
#42443=EDGE_LOOP ( 'NONE', ( #39861, #13439, #36605, #357, #17040, #28841 ) ) ;
#42448=EDGE_CURVE ( 'NONE', #39697, #7984, #23036, .T. ) ;
#42455=EDGE_CURVE ( 'NONE', #39212, #2677, #20118, .T. ) ;
#42467=CARTESIAN_POINT ( 'NONE',  ( -26.63011601220122060, -513.1383975375929367, -369.9999999999999432 ) ) ;
#42476=ADVANCED_FACE ( 'NONE', ( #612 ), #35019, .F. ) ;
#42516=ORIENTED_EDGE ( 'NONE', *, *, #30332, .T. ) ;
#42519=CYLINDRICAL_SURFACE ( 'NONE', #38085, 12.00000000000001066 ) ;
#42573=VECTOR ( 'NONE', #5877, 1000.000000000000114 ) ;
#42577=ORIENTED_EDGE ( 'NONE', *, *, #16352, .T. ) ;
#42615=CARTESIAN_POINT ( 'NONE',  ( 786.4999999999993179, 26.27639943461401018, 900.0000000000001137 ) ) ;
#42618=ORIENTED_EDGE ( 'NONE', *, *, #23553, .F. ) ;
#42624=ORIENTED_EDGE ( 'NONE', *, *, #18364, .F. ) ;
#42631=ORIENTED_EDGE ( 'NONE', *, *, #6342, .T. ) ;
#42641=ORIENTED_EDGE ( 'NONE', *, *, #20155, .T. ) ;
#42643=DIRECTION ( 'NONE',  ( 0.000000000000000000, 0.000000000000000000, -1.000000000000000000 ) ) ;
#42650=DIRECTION ( 'NONE',  ( 0.000000000000000000, 0.3826834323650836200, 0.9238795325112892920 ) ) ;
#42662=DIRECTION ( 'NONE',  ( -1.000000000000000000, 0.000000000000000000, 0.000000000000000000 ) ) ;
#42666=VECTOR ( 'NONE', #14573, 1000.000000000000000 ) ;
#42668=CARTESIAN_POINT ( 'NONE',  ( -786.4999999999993179, -544.8427095258973623, -350.0000000000000000 ) ) ;
#42697=EDGE_CURVE ( 'NONE', #16430, #23506, #36378, .T. ) ;
#42763=LINE ( 'NONE', #36513, #1376 ) ;
#42769=ADVANCED_FACE ( 'NONE', ( #1289 ), #1499, .F. ) ;
#42787=ORIENTED_EDGE ( 'NONE', *, *, #23553, .T. ) ;
#42832=CARTESIAN_POINT ( 'NONE',  ( 786.4999999999993179, -513.1383975375929367, -349.9999999999999432 ) ) ;
#42839=DIRECTION ( 'NONE',  ( -1.000000000000000000, -0.000000000000000000, -0.000000000000000000 ) ) ;
#42847=ORIENTED_EDGE ( 'NONE', *, *, #16352, .F. ) ;
#42853=DIRECTION ( 'NONE',  ( 0.000000000000000000, 0.000000000000000000, 1.000000000000000000 ) ) ;
#42871=CARTESIAN_POINT ( 'NONE',  ( -26.63011601220122060, -544.8427095258973623, -369.9999999999999432 ) ) ;
#42877=CARTESIAN_POINT ( 'NONE',  ( -746.4999999999993179, -365.3551492539851893, -18.13243251470705886 ) ) ;
#42883=CARTESIAN_POINT ( 'NONE',  ( 786.4999999999993179, -513.1383975375929367, -369.9999999999999432 ) ) ;
#42893=EDGE_LOOP ( 'NONE', ( #11499, #43186, #36715, #26327, #10470, #5674, #20, #24084 ) ) ;
#42909=PLANE ( 'NONE',  #14745 ) ;
#42931=DIRECTION ( 'NONE',  ( 1.000000000000000000, -0.000000000000000000, -0.000000000000000000 ) ) ;
#42983=AXIS2_PLACEMENT_3D ( 'NONE', #18350, #17878, #22234 ) ;
#43039=DIRECTION ( 'NONE',  ( 1.000000000000000000, -0.000000000000000000, -0.000000000000000000 ) ) ;
#43045=ADVANCED_FACE ( 'NONE', ( #8011, #4529, #25769 ), #39881, .T. ) ;
#43056=FACE_OUTER_BOUND ( 'NONE', #36607, .T. ) ;
#43087=LINE ( 'NONE', #25760, #43244 ) ;
#43109=DIRECTION ( 'NONE',  ( 0.000000000000000000, 0.000000000000000000, 1.000000000000000000 ) ) ;
#43134=ORIENTED_EDGE ( 'NONE', *, *, #29222, .T. ) ;
#43151=VECTOR ( 'NONE', #43039, 1000.000000000000000 ) ;
#43162=DIRECTION ( 'NONE',  ( -1.000000000000000000, 0.000000000000000000, 0.000000000000000000 ) ) ;
#43174=ORIENTED_EDGE ( 'NONE', *, *, #18364, .T. ) ;
#43180=AXIS2_PLACEMENT_3D ( 'NONE', #12746, #4922, #26825 ) ;
#43186=ORIENTED_EDGE ( 'NONE', *, *, #29862, .F. ) ;
#43196=EDGE_LOOP ( 'NONE', ( #14874, #36192 ) ) ;
#43200=DIRECTION ( 'NONE',  ( 1.000000000000000000, -0.000000000000000000, -0.000000000000000000 ) ) ;
#43244=VECTOR ( 'NONE', #35932, 1000.000000000000000 ) ;
#43251=VERTEX_POINT ( 'NONE', #16505 ) ;
#43262=EDGE_CURVE ( 'NONE', #17108, #5117, #12803, .T. ) ;
#43271=CARTESIAN_POINT ( 'NONE',  ( 1007.605605532488426, -30.07539427629357576, 756.1153575698151599 ) ) ;
#43278=AXIS2_PLACEMENT_3D ( 'NONE', #22507, #40744, #1490 ) ;
#43286=LINE ( 'NONE', #21577, #19573 ) ;
#43293=EDGE_CURVE ( 'NONE', #19543, #34761, #8894, .T. ) ;
#43312=DIRECTION ( 'NONE',  ( -0.000000000000000000, 0.000000000000000000, 1.000000000000000000 ) ) ;
#43333=DIRECTION ( 'NONE',  ( 1.000000000000000000, -0.000000000000000000, -0.000000000000000000 ) ) ;
#43339=DIRECTION ( 'NONE',  ( 0.000000000000000000, 1.000000000000000000, -0.000000000000000000 ) ) ;
#43340=LINE ( 'NONE', #39205, #12423 ) ;
#43356=ORIENTED_EDGE ( 'NONE', *, *, #4722, .F. ) ;
#43372=EDGE_CURVE ( 'NONE', #463, #38191, #12756, .T. ) ;
#43377=DIRECTION ( 'NONE',  ( -0.000000000000000000, -0.3826834323650836756, -0.9238795325112892920 ) ) ;
#43380=LINE ( 'NONE', #25814, #17480 ) ;
#43406=CARTESIAN_POINT ( 'NONE',  ( -26.63011601220122060, -496.5085659523897448, -356.8883017825714319 ) ) ;
#43422=ORIENTED_EDGE ( 'NONE', *, *, #35409, .F. ) ;
#43427=LINE ( 'NONE', #18721, #6902 ) ;
#43446=DIRECTION ( 'NONE',  ( -1.000000000000000000, 0.000000000000000000, 0.000000000000000000 ) ) ;
#43472=ORIENTED_EDGE ( 'NONE', *, *, #29773, .T. ) ;
#43479=CARTESIAN_POINT ( 'NONE',  ( -37.63011601220122770, -563.3203001761230553, -342.3463313526983143 ) ) ;
#43522=EDGE_LOOP ( 'NONE', ( #9710, #27437, #25240, #7251 ) ) ;
#43560=ADVANCED_FACE ( 'NONE', ( #27575 ), #28895, .F. ) ;
#43564=DIRECTION ( 'NONE',  ( 0.000000000000000000, 0.000000000000000000, 1.000000000000000000 ) ) ;
#43573=ORIENTED_EDGE ( 'NONE', *, *, #169, .F. ) ;
#43588=EDGE_CURVE ( 'NONE', #32812, #18154, #2442, .T. ) ;
#43593=ADVANCED_FACE ( 'NONE', ( #13959, #25661, #38436 ), #36059, .T. ) ;
#43603=CARTESIAN_POINT ( 'NONE',  ( 1007.605605532488426, -110.5936016518798652, 750.6326042729449455 ) ) ;
#43608=ORIENTED_EDGE ( 'NONE', *, *, #21836, .F. ) ;
#43611=ADVANCED_FACE ( 'NONE', ( #24553 ), #20641, .T. ) ;
#43616=EDGE_LOOP ( 'NONE', ( #8418, #38288, #7248, #18873 ) ) ;
#43666=CARTESIAN_POINT ( 'NONE',  ( -746.4999999999993179, -365.3551492539851893, -28.13243251470704109 ) ) ;
#43682=LINE ( 'NONE', #40009, #32316 ) ;
#43697=CARTESIAN_POINT ( 'NONE',  ( -26.63011601220122060, -512.9681489794448908, -339.9999999999999432 ) ) ;
#43700=CARTESIAN_POINT ( 'NONE',  ( -26.63011601220122060, -563.3203001761230553, -342.3463313526983143 ) ) ;
#43725=ORIENTED_EDGE ( 'NONE', *, *, #35171, .T. ) ;
#43730=EDGE_LOOP ( 'NONE', ( #18832, #6498 ) ) ;
#43743=CARTESIAN_POINT ( 'NONE',  ( -26.63011601220122060, -513.1383975375929367, -349.9999999999999432 ) ) ;
#43757=DIRECTION ( 'NONE',  ( 0.000000000000000000, 0.9238795325112891810, -0.3826834323650838421 ) ) ;
#43778=VECTOR ( 'NONE', #2413, 1000.000000000000000 ) ;
#43798=PLANE ( 'NONE',  #23277 ) ;
#43812=ORIENTED_EDGE ( 'NONE', *, *, #11429, .T. ) ;
#43829=VECTOR ( 'NONE', #18631, 1000.000000000000114 ) ;
#43843=AXIS2_PLACEMENT_3D ( 'NONE', #5833, #12087, #9060 ) ;
#43884=AXIS2_PLACEMENT_3D ( 'NONE', #503, #14830, #10906 ) ;
#43890=AXIS2_PLACEMENT_3D ( 'NONE', #29011, #29676, #18850 ) ;
#43963=PLANE ( 'NONE',  #26363 ) ;
#43968=( LENGTH_UNIT ( ) NAMED_UNIT ( * ) SI_UNIT ( .MILLI., .METRE. ) );
#43991=DIRECTION ( 'NONE',  ( 0.000000000000000000, 0.000000000000000000, -1.000000000000000000 ) ) ;
#44015=VERTEX_POINT ( 'NONE', #8954 ) ;
#44019=CARTESIAN_POINT ( 'NONE',  ( -39.63011601220123481, -544.8427095258973623, -369.9999999999999432 ) ) ;
#44022=AXIS2_PLACEMENT_3D ( 'NONE', #38550, #7844, #14544 ) ;
#44036=LINE ( 'NONE', #5026, #4119 ) ;
#44060=EDGE_CURVE ( 'NONE', #4703, #45720, #39358, .T. ) ;
#44062=ORIENTED_EDGE ( 'NONE', *, *, #988, .T. ) ;
#44082=ORIENTED_EDGE ( 'NONE', *, *, #20764, .T. ) ;
#44153=CYLINDRICAL_SURFACE ( 'NONE', #13792, 9.999999999999980460 ) ;
#44162=EDGE_CURVE ( 'NONE', #9315, #1111, #30495, .T. ) ;
#44167=CYLINDRICAL_SURFACE ( 'NONE', #24030, 19.99999999999990763 ) ;
#44169=DIRECTION ( 'NONE',  ( 0.000000000000000000, -0.3826834323650837866, -0.9238795325112891810 ) ) ;
#44193=EDGE_LOOP ( 'NONE', ( #6898, #34068 ) ) ;
#44196=ORIENTED_EDGE ( 'NONE', *, *, #45351, .F. ) ;
#44197=CARTESIAN_POINT ( 'NONE',  ( -784.4999999999993179, -359.5698779088871788, -26.28906389436296109 ) ) ;
#44209=FACE_OUTER_BOUND ( 'NONE', #30893, .T. ) ;
#44213=DIRECTION ( 'NONE',  ( -1.000000000000000000, -0.000000000000000000, -0.000000000000000000 ) ) ;
#44223=DIRECTION ( 'NONE',  ( 0.000000000000000000, -0.3826834323650838976, -0.9238795325112892920 ) ) ;
#44238=DIRECTION ( 'NONE',  ( -1.000000000000000000, -0.000000000000000000, -0.000000000000000000 ) ) ;
#44247=ORIENTED_EDGE ( 'NONE', *, *, #42455, .T. ) ;
#44252=CARTESIAN_POINT ( 'NONE',  ( 784.4999999999993179, -365.3551492539851893, -8.132432514707076621 ) ) ;
#44292=ORIENTED_EDGE ( 'NONE', *, *, #16579, .F. ) ;
#44312=ORIENTED_EDGE ( 'NONE', *, *, #35742, .T. ) ;
#44337=DIRECTION ( 'NONE',  ( -1.000000000000000000, -0.000000000000000000, 0.000000000000000000 ) ) ;
#44366=ORIENTED_EDGE ( 'NONE', *, *, #42448, .F. ) ;
#44390=VECTOR ( 'NONE', #4980, 1000.000000000000000 ) ;
#44391=PLANE ( 'NONE',  #43180 ) ;
#44413=AXIS2_PLACEMENT_3D ( 'NONE', #18503, #3499, #21491 ) ;
#44425=ORIENTED_EDGE ( 'NONE', *, *, #32862, .F. ) ;
#44431=DIRECTION ( 'NONE',  ( 1.000000000000000000, -0.000000000000000000, -0.000000000000000000 ) ) ;
#44478=VERTEX_POINT ( 'NONE', #2937 ) ;
#44484=AXIS2_PLACEMENT_3D ( 'NONE', #2875, #16276, #30355 ) ;
#44499=ADVANCED_FACE ( 'NONE', ( #17024 ), #38495, .F. ) ;
#44500=( GEOMETRIC_REPRESENTATION_CONTEXT ( 3 ) GLOBAL_UNCERTAINTY_ASSIGNED_CONTEXT ( ( #17326 ) ) GLOBAL_UNIT_ASSIGNED_CONTEXT ( ( #40357, #5437, #33629 ) ) REPRESENTATION_CONTEXT ( 'NONE', 'WORKASPACE' ) );
#44556=ORIENTED_EDGE ( 'NONE', *, *, #37672, .T. ) ;
#44569=AXIS2_PLACEMENT_3D ( 'NONE', #36017, #35781, #32328 ) ;
#44571=CARTESIAN_POINT ( 'NONE',  ( -786.4999999999993179, -110.5936016518799221, 750.6326042729449455 ) ) ;
#44599=DIRECTION ( 'NONE',  ( -1.000000000000000000, -0.000000000000000000, -0.000000000000000000 ) ) ;
#44617=DIRECTION ( 'NONE',  ( 0.000000000000000000, 0.3826834323650836200, 0.9238795325112892920 ) ) ;
#44627=FACE_BOUND ( 'NONE', #44193, .T. ) ;
#44637=DIRECTION ( 'NONE',  ( 1.000000000000000000, 0.000000000000000000, 0.000000000000000000 ) ) ;
#44647=ORIENTED_EDGE ( 'NONE', *, *, #45466, .F. ) ;
#44673=VECTOR ( 'NONE', #35004, 1000.000000000000114 ) ;
#44691=AXIS2_PLACEMENT_3D ( 'NONE', #30343, #30814, #31034 ) ;
#44694=LINE ( 'NONE', #34053, #15864 ) ;
#44718=ORIENTED_EDGE ( 'NONE', *, *, #6964, .F. ) ;
#44728=CIRCLE ( 'NONE', #24061, 10.00000000000000888 ) ;
#44733=ADVANCED_FACE ( 'NONE', ( #18857 ), #11470, .T. ) ;
#44749=CARTESIAN_POINT ( 'NONE',  ( -26.63011601220122060, -494.6608068873671300, -357.6536686473015720 ) ) ;
#44756=DIRECTION ( 'NONE',  ( 0.000000000000000000, 0.000000000000000000, -1.000000000000000000 ) ) ;
#44761=DIRECTION ( 'NONE',  ( 1.000000000000000000, 0.000000000000000000, 0.000000000000000000 ) ) ;
#44775=PLANE ( 'NONE',  #34374 ) ;
#44784=ADVANCED_FACE ( 'NONE', ( #384 ), #10784, .T. ) ;
#44853=LINE ( 'NONE', #19906, #24114 ) ;
#44860=LINE ( 'NONE', #9741, #39246 ) ;
#44865=CARTESIAN_POINT ( 'NONE',  ( -773.4999999999993179, -365.3551492539851893, -8.132432514707076621 ) ) ;
#44866=VECTOR ( 'NONE', #38057, 1000.000000000000000 ) ;
#44868=CARTESIAN_POINT ( 'NONE',  ( -26.63011601220122060, -365.3551492539851893, -18.13243251470705886 ) ) ;
#44872=CARTESIAN_POINT ( 'NONE',  ( -39.63011601220123481, -110.5936016518799221, 750.6326042729449455 ) ) ;
#44892=VERTEX_POINT ( 'NONE', #1058 ) ;
#44893=SHAPE_REPRESENTATION_RELATIONSHIP ( 'NONE' , 'NONE' ,  #4721, #39222 ) ;
#44899=CIRCLE ( 'NONE', #32381, 9.999999999999982236 ) ;
#44937=DIRECTION ( 'NONE',  ( -1.000000000000000000, -0.000000000000000000, -0.000000000000000000 ) ) ;
#44956=VERTEX_POINT ( 'NONE', #42871 ) ;
#44996=VERTEX_POINT ( 'NONE', #5658 ) ;
#45002=ORIENTED_EDGE ( 'NONE', *, *, #36874, .T. ) ;
#45039=EDGE_CURVE ( 'NONE', #11223, #2103, #34054, .T. ) ;
#45042=CARTESIAN_POINT ( 'NONE',  ( 786.4999999999993179, -544.8427095258973623, -350.0000000000000000 ) ) ;
#45051=EDGE_CURVE ( 'NONE', #22547, #11840, #12141, .T. ) ;
#45083=ORIENTED_EDGE ( 'NONE', *, *, #11477, .T. ) ;
#45087=ADVANCED_FACE ( 'NONE', ( #16513 ), #19079, .T. ) ;
#45118=ORIENTED_EDGE ( 'NONE', *, *, #1487, .T. ) ;
#45123=ORIENTED_EDGE ( 'NONE', *, *, #22178, .T. ) ;
#45148=( LENGTH_UNIT ( ) NAMED_UNIT ( * ) SI_UNIT ( .MILLI., .METRE. ) );
#45169=CARTESIAN_POINT ( 'NONE',  ( 773.4999999999993179, -110.5936016518799221, 750.6326042729449455 ) ) ;
#45192=CARTESIAN_POINT ( 'NONE',  ( 786.4999999999993179, -544.8427095258973623, -369.9999999999999432 ) ) ;
#45196=DIRECTION ( 'NONE',  ( -1.000000000000000000, -0.000000000000000000, -0.000000000000000000 ) ) ;
#45248=ORIENTED_EDGE ( 'NONE', *, *, #44060, .T. ) ;
#45283=VECTOR ( 'NONE', #9360, 1000.000000000000000 ) ;
#45316=EDGE_CURVE ( 'NONE', #44956, #4358, #40764, .T. ) ;
#45342=EDGE_CURVE ( 'NONE', #19960, #39647, #37152, .T. ) ;
#45351=EDGE_CURVE ( 'NONE', #7814, #69, #27821, .T. ) ;
#45352=EDGE_LOOP ( 'NONE', ( #19157, #29433, #23065, #26758 ) ) ;
#45370=CARTESIAN_POINT ( 'NONE',  ( 786.4999999999993179, -292.9981031064102126, 121.3637880562633171 ) ) ;
#45393=CIRCLE ( 'NONE', #3315, 19.99999999999990763 ) ;
#45415=ORIENTED_EDGE ( 'NONE', *, *, #35997, .T. ) ;
#45421=LINE ( 'NONE', #30867, #44673 ) ;
#45436=CARTESIAN_POINT ( 'NONE',  ( -28.63011601220122415, -365.3551492539851893, -18.13243251470705886 ) ) ;
#45454=CARTESIAN_POINT ( 'NONE',  ( 786.4999999999993179, -365.3551492539851893, -18.13243251470705886 ) ) ;
#45466=EDGE_CURVE ( 'NONE', #2958, #40161, #23649, .T. ) ;
#45475=VECTOR ( 'NONE', #19957, 1000.000000000000000 ) ;
#45502=DIRECTION ( 'NONE',  ( 0.000000000000000000, -0.9238795325112835188, 0.3826834323650978309 ) ) ;
#45512=CIRCLE ( 'NONE', #25591, 9.999999999999982236 ) ;
#45529=VECTOR ( 'NONE', #7369, 1000.000000000000000 ) ;
#45546=PLANE ( 'NONE',  #10718 ) ;
#45565=EDGE_CURVE ( 'NONE', #4358, #44996, #26109, .T. ) ;
#45572=LINE ( 'NONE', #37937, #41718 ) ;
#45611=CARTESIAN_POINT ( 'NONE',  ( 775.4999999999993179, -365.3551492539851893, -18.13243251470705886 ) ) ;
#45612=DIRECTION ( 'NONE',  ( 1.000000000000000000, -0.000000000000000000, -0.000000000000000000 ) ) ;
#45615=CARTESIAN_POINT ( 'NONE',  ( -784.4999999999993179, -501.1515549466498669, -368.0974687824633520 ) ) ;
#45642=VERTEX_POINT ( 'NONE', #44197 ) ;
#45651=ORIENTED_EDGE ( 'NONE', *, *, #42114, .F. ) ;
#45669=DIRECTION ( 'NONE',  ( 0.000000000000000000, 0.000000000000000000, 1.000000000000000000 ) ) ;
#45674=AXIS2_PLACEMENT_3D ( 'NONE', #8580, #11592, #8343 ) ;
#45679=LINE ( 'NONE', #42196, #4751 ) ;
#45680=CARTESIAN_POINT ( 'NONE',  ( 786.4999999999993179, -512.9681489794448908, -339.9999999999999432 ) ) ;
#45692=DIRECTION ( 'NONE',  ( -1.000000000000000000, 0.000000000000000000, 0.000000000000000000 ) ) ;
#45695=EDGE_LOOP ( 'NONE', ( #36596, #42577 ) ) ;
#45699=ORIENTED_EDGE ( 'NONE', *, *, #20069, .T. ) ;
#45720=VERTEX_POINT ( 'NONE', #12557 ) ;
#45752=COLOUR_RGB('Sky Blue',0.24,0.69,0.87);
#45753=FILL_AREA_STYLE_COLOUR('',#45752);
#45754=FILL_AREA_STYLE('',(#45753));
#45755=SURFACE_STYLE_FILL_AREA(#45754);
#45756=SURFACE_SIDE_STYLE('',(#45755));
#45757=SURFACE_STYLE_USAGE(.BOTH.,#45756);
#45758=PRESENTATION_STYLE_ASSIGNMENT((#45757));
ENDSEC;
END-ISO-10303-21;
